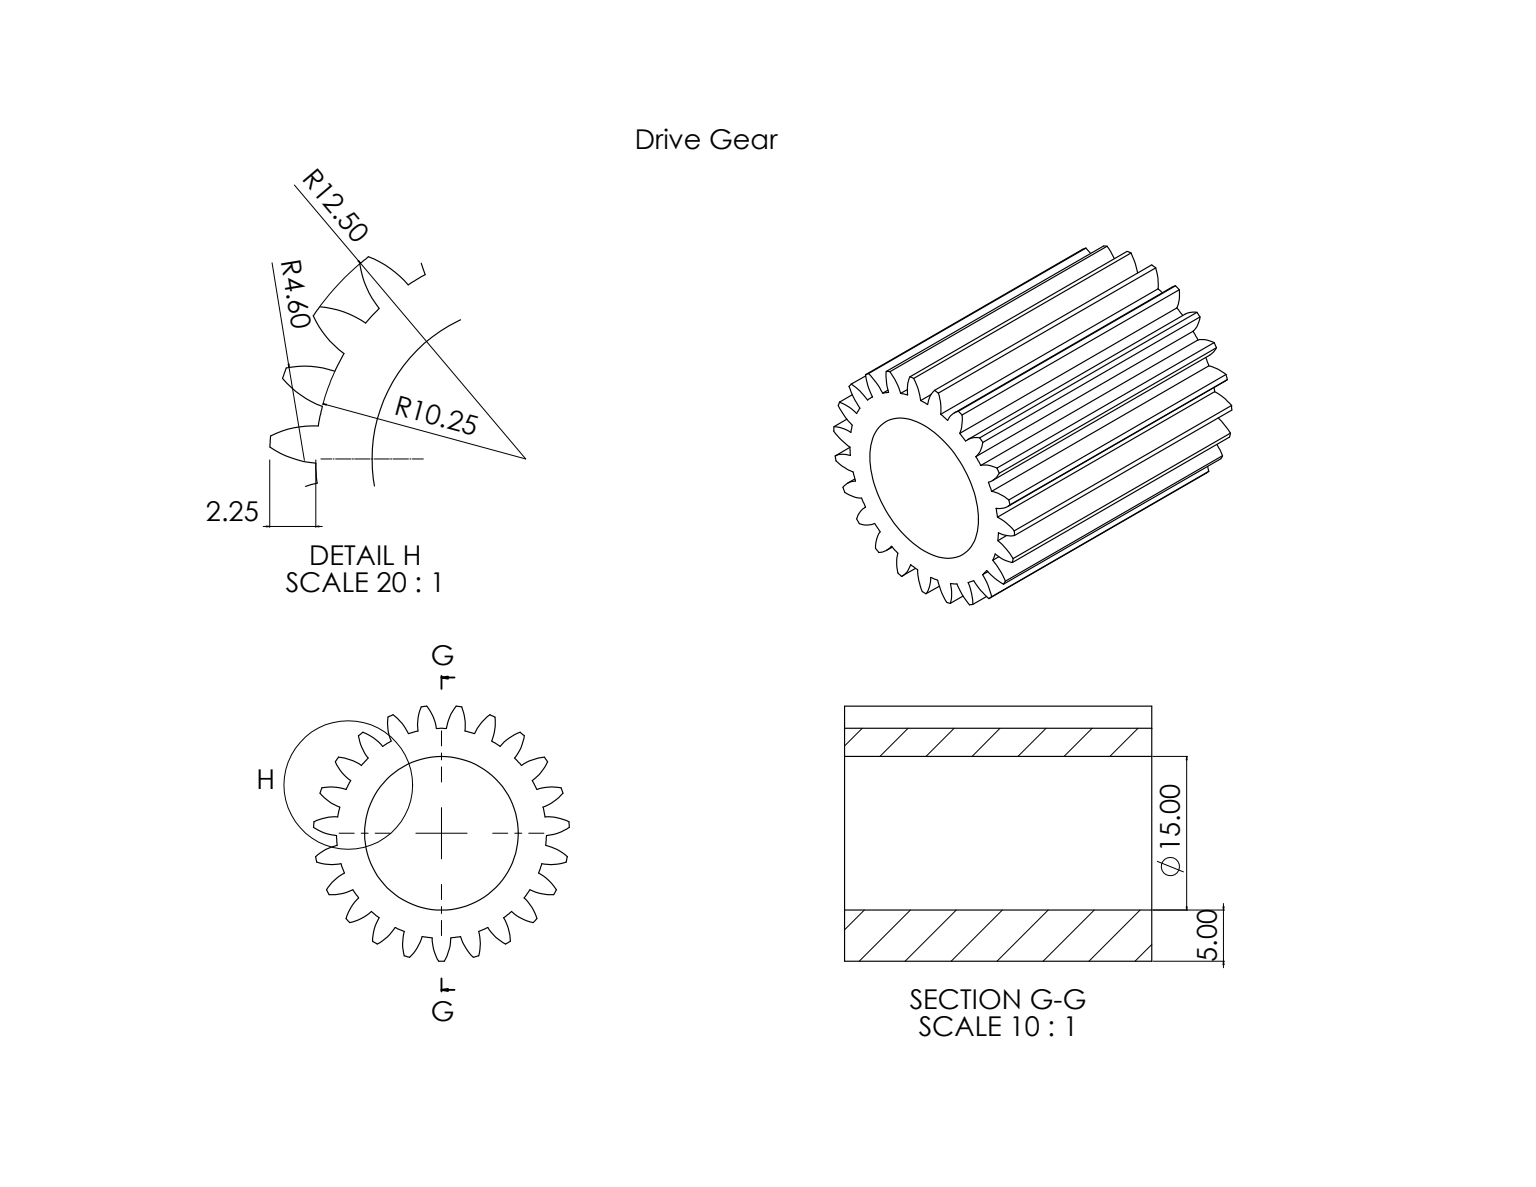
ISO-10303-21;
HEADER;
FILE_DESCRIPTION (('STEP AP214'),
    '1' );
FILE_NAME ('Drive Gear.step',
    '2026-10-21T18:33:49',
    ( '' ),
    ( '' ),
    'SwSTEP 2.0',
    'SolidWorks 2025',
    '' );
FILE_SCHEMA (( 'AUTOMOTIVE_DESIGN' ));
ENDSEC;

DATA;
#7=CIRCLE ( 'NONE', #9259, 4.600000000000006750 ) ;
#13=CIRCLE ( 'NONE', #606, 12.50000000000001776 ) ;
#15=ADVANCED_FACE ( 'NONE', ( #8489 ), #16983, .T. ) ;
#16=DIRECTION ( 'NONE',  ( -5.204170427930409450E-16, 0.000000000000000000, 1.000000000000000000 ) ) ;
#17=ORIENTED_EDGE ( 'NONE', *, *, #6060, .F. ) ;
#19=ADVANCED_FACE ( 'NONE', ( #15595 ), #11103, .T. ) ;
#20=ADVANCED_FACE ( 'NONE', ( #8576 ), #7163, .T. ) ;
#21=CARTESIAN_POINT ( 'NONE',  ( -67.50540723371459251, 87.07303407725210320, 15.00000000000006928 ) ) ;
#30=EDGE_LOOP ( 'NONE', ( #4057, #14157, #6420, #5551 ) ) ;
#37=EDGE_LOOP ( 'NONE', ( #6433, #6306, #4816, #14039 ) ) ;
#40=ORIENTED_EDGE ( 'NONE', *, *, #16480, .F. ) ;
#42=DIRECTION ( 'NONE',  ( -1.000000000000000000, 5.416250486023790304E-15, 1.692578276882434470E-16 ) ) ;
#50=ORIENTED_EDGE ( 'NONE', *, *, #8115, .F. ) ;
#51=AXIS2_PLACEMENT_3D ( 'NONE', #16170, #17306, #13379 ) ;
#53=ORIENTED_EDGE ( 'NONE', *, *, #16344, .F. ) ;
#56=AXIS2_PLACEMENT_3D ( 'NONE', #11345, #9554, #17037 ) ;
#58=DIRECTION ( 'NONE',  ( -1.000000000000000000, 0.000000000000000000, 1.156482317317869999E-16 ) ) ;
#61=CARTESIAN_POINT ( 'NONE',  ( -44.89980253466632831, 81.41924511788819530, 15.00000000000006928 ) ) ;
#62=DIRECTION ( 'NONE',  ( 1.000000000000000000, 0.000000000000000000, 5.077734830647299712E-16 ) ) ;
#70=VERTEX_POINT ( 'NONE', #417 ) ;
#71=CIRCLE ( 'NONE', #16786, 10.24900000000000055 ) ;
#72=VECTOR ( 'NONE', #8079, 1000.000000000000000 ) ;
#75=CARTESIAN_POINT ( 'NONE',  ( -59.35080917176598092, 94.79374675277695417, -15.00000000000001421 ) ) ;
#83=AXIS2_PLACEMENT_3D ( 'NONE', #305, #8649, #15842 ) ;
#86=CARTESIAN_POINT ( 'NONE',  ( -67.32681558843928826, 84.01587117655452630, 15.00000000000006928 ) ) ;
#92=FACE_OUTER_BOUND ( 'NONE', #4705, .T. ) ;
#97=EDGE_LOOP ( 'NONE', ( #14559, #13719, #17905, #14362 ) ) ;
#98=VECTOR ( 'NONE', #835, 1000.000000000000000 ) ;
#104=VECTOR ( 'NONE', #14107, 1000.000000000000000 ) ;
#113=VERTEX_POINT ( 'NONE', #1813 ) ;
#114=CARTESIAN_POINT ( 'NONE',  ( -57.08002265617300708, 84.22855780814606419, 15.00000000000006928 ) ) ;
#145=EDGE_LOOP ( 'NONE', ( #17261, #13971, #8851, #5219 ) ) ;
#147=DIRECTION ( 'NONE',  ( 1.156482317317869999E-16, 0.000000000000000000, 1.000000000000000000 ) ) ;
#149=ORIENTED_EDGE ( 'NONE', *, *, #11735, .T. ) ;
#150=EDGE_CURVE ( 'NONE', #4219, #3665, #3494, .T. ) ;
#154=AXIS2_PLACEMENT_3D ( 'NONE', #13342, #6302, #517 ) ;
#169=CARTESIAN_POINT ( 'NONE',  ( -59.35080917176598092, 94.79374675277695417, 15.00000000000006928 ) ) ;
#175=DIRECTION ( 'NONE',  ( 1.000000000000000000, 0.000000000000000000, 0.000000000000000000 ) ) ;
#179=DIRECTION ( 'NONE',  ( 1.000000000000000000, 0.000000000000000000, 5.551115123125780730E-16 ) ) ;
#187=DIRECTION ( 'NONE',  ( -5.204170427930409450E-16, 0.000000000000000000, 1.000000000000000000 ) ) ;
#191=DIRECTION ( 'NONE',  ( 1.156482317317869999E-16, 0.000000000000000000, 1.000000000000000000 ) ) ;
#195=CYLINDRICAL_SURFACE ( 'NONE', #16432, 4.599999999999999645 ) ;
#197=VERTEX_POINT ( 'NONE', #9569 ) ;
#200=ORIENTED_EDGE ( 'NONE', *, *, #18072, .T. ) ;
#201=DIRECTION ( 'NONE',  ( -1.000000000000000000, 2.331468351712825579E-14, 1.387778780781443703E-16 ) ) ;
#209=DIRECTION ( 'NONE',  ( 1.156482317317869999E-16, 0.000000000000000000, 1.000000000000000000 ) ) ;
#210=ORIENTED_EDGE ( 'NONE', *, *, #16102, .F. ) ;
#216=DIRECTION ( 'NONE',  ( 0.000000000000000000, 0.000000000000000000, 1.000000000000000000 ) ) ;
#220=ORIENTED_EDGE ( 'NONE', *, *, #11450, .F. ) ;
#237=CYLINDRICAL_SURFACE ( 'NONE', #286, 4.599999999999999645 ) ;
#249=CYLINDRICAL_SURFACE ( 'NONE', #1928, 10.24900000000000766 ) ;
#253=EDGE_LOOP ( 'NONE', ( #10457, #6808, #9246, #11912 ) ) ;
#256=DIRECTION ( 'NONE',  ( 0.000000000000000000, 0.000000000000000000, 1.000000000000000000 ) ) ;
#265=DIRECTION ( 'NONE',  ( 0.000000000000000000, 0.000000000000000000, 1.000000000000000000 ) ) ;
#272=CARTESIAN_POINT ( 'NONE',  ( -67.13262496892538422, 91.65790412808873100, -167.1454815528550739 ) ) ;
#274=VERTEX_POINT ( 'NONE', #11460 ) ;
#286=AXIS2_PLACEMENT_3D ( 'NONE', #17181, #15858, #14286 ) ;
#295=DIRECTION ( 'NONE',  ( 1.000000000000000000, 0.000000000000000000, 3.771137991253934490E-16 ) ) ;
#297=EDGE_CURVE ( 'NONE', #9307, #9072, #17170, .T. ) ;
#304=VECTOR ( 'NONE', #7741, 1000.000000000000000 ) ;
#305=CARTESIAN_POINT ( 'NONE',  ( -56.26901274438541378, 73.45256821284058901, -15.00000000000001421 ) ) ;
#309=EDGE_CURVE ( 'NONE', #9564, #16752, #11785, .T. ) ;
#311=EDGE_CURVE ( 'NONE', #17138, #8972, #12775, .T. ) ;
#319=FACE_BOUND ( 'NONE', #1203, .T. ) ;
#321=EDGE_LOOP ( 'NONE', ( #11496, #14503 ) ) ;
#328=CYLINDRICAL_SURFACE ( 'NONE', #16782, 4.599999999999999645 ) ;
#329=DIRECTION ( 'NONE',  ( 1.156482317317869999E-16, 0.000000000000000000, 1.000000000000000000 ) ) ;
#332=AXIS2_PLACEMENT_3D ( 'NONE', #14799, #4971, #14887 ) ;
#340=ADVANCED_FACE ( 'NONE', ( #13312 ), #13217, .T. ) ;
#348=CARTESIAN_POINT ( 'NONE',  ( -65.94558993203320085, 89.37090336996871542, -167.1454815528550739 ) ) ;
#351=ORIENTED_EDGE ( 'NONE', *, *, #16581, .T. ) ;
#352=DIRECTION ( 'NONE',  ( 1.000000000000000000, 0.000000000000000000, 0.000000000000000000 ) ) ;
#353=AXIS2_PLACEMENT_3D ( 'NONE', #9432, #13643, #6427 ) ;
#362=EDGE_CURVE ( 'NONE', #16861, #16195, #8816, .T. ) ;
#363=LINE ( 'NONE', #13186, #2716 ) ;
#369=ORIENTED_EDGE ( 'NONE', *, *, #4474, .F. ) ;
#370=ORIENTED_EDGE ( 'NONE', *, *, #2385, .F. ) ;
#402=AXIS2_PLACEMENT_3D ( 'NONE', #10590, #6260, #12088 ) ;
#415=VERTEX_POINT ( 'NONE', #17506 ) ;
#417=CARTESIAN_POINT ( 'NONE',  ( -50.35400969968294049, 73.69239390902568232, 15.00000000000006928 ) ) ;
#428=CARTESIAN_POINT ( 'NONE',  ( -57.08002265617300708, 84.22855780814606419, -167.1454815528550739 ) ) ;
#431=CARTESIAN_POINT ( 'NONE',  ( -67.77554565888843285, 85.77305660501664875, 15.00000000000006928 ) ) ;
#434=CIRCLE ( 'NONE', #4026, 12.50000000000001066 ) ;
#435=ORIENTED_EDGE ( 'NONE', *, *, #15098, .T. ) ;
#436=VECTOR ( 'NONE', #9546, 1000.000000000000000 ) ;
#439=CARTESIAN_POINT ( 'NONE',  ( -63.80603561266293156, 73.69239390902558284, -167.1454815528550739 ) ) ;
#440=EDGE_CURVE ( 'NONE', #16158, #9400, #4619, .T. ) ;
#445=DIRECTION ( 'NONE',  ( 0.000000000000000000, 0.000000000000000000, 1.000000000000000000 ) ) ;
#447=CIRCLE ( 'NONE', #16265, 4.599999999999999645 ) ;
#458=ORIENTED_EDGE ( 'NONE', *, *, #15095, .T. ) ;
#465=AXIS2_PLACEMENT_3D ( 'NONE', #15310, #8209, #13925 ) ;
#466=EDGE_CURVE ( 'NONE', #2633, #113, #1358, .T. ) ;
#469=EDGE_CURVE ( 'NONE', #3406, #8935, #14485, .T. ) ;
#472=DIRECTION ( 'NONE',  ( 1.000000000000000000, 0.000000000000000000, 0.000000000000000000 ) ) ;
#475=DIRECTION ( 'NONE',  ( 1.156482317317869999E-16, 0.000000000000000000, 1.000000000000000000 ) ) ;
#477=ORIENTED_EDGE ( 'NONE', *, *, #4383, .F. ) ;
#489=EDGE_CURVE ( 'NONE', #6937, #4200, #6985, .T. ) ;
#493=ORIENTED_EDGE ( 'NONE', *, *, #10731, .F. ) ;
#498=CARTESIAN_POINT ( 'NONE',  ( -57.08002265617300708, 84.22855780814606419, -15.00000000000001421 ) ) ;
#502=FACE_OUTER_BOUND ( 'NONE', #5462, .T. ) ;
#511=ORIENTED_EDGE ( 'NONE', *, *, #14433, .F. ) ;
#514=CARTESIAN_POINT ( 'NONE',  ( -57.08002265617300708, 84.22855780814606419, 15.00000000000006928 ) ) ;
#517=DIRECTION ( 'NONE',  ( -1.000000000000000000, -3.016910393003147592E-15, 0.000000000000000000 ) ) ;
#518=DIRECTION ( 'NONE',  ( 1.000000000000000000, 0.000000000000000000, 0.000000000000000000 ) ) ;
#519=ORIENTED_EDGE ( 'NONE', *, *, #11473, .F. ) ;
#522=DIRECTION ( 'NONE',  ( 0.000000000000000000, 0.000000000000000000, 1.000000000000000000 ) ) ;
#526=DIRECTION ( 'NONE',  ( 0.000000000000000000, 0.000000000000000000, 1.000000000000000000 ) ) ;
#528=EDGE_LOOP ( 'NONE', ( #8354, #7996, #14007, #17143 ) ) ;
#538=VERTEX_POINT ( 'NONE', #3755 ) ;
#539=EDGE_CURVE ( 'NONE', #1636, #14316, #3687, .T. ) ;
#544=AXIS2_PLACEMENT_3D ( 'NONE', #10480, #10583, #14958 ) ;
#548=EDGE_CURVE ( 'NONE', #15230, #8556, #6062, .T. ) ;
#563=DIRECTION ( 'NONE',  ( 0.000000000000000000, 0.000000000000000000, 1.000000000000000000 ) ) ;
#566=ADVANCED_FACE ( 'NONE', ( #8045 ), #954, .T. ) ;
#567=DIRECTION ( 'NONE',  ( 1.000000000000000000, 0.000000000000000000, 5.077734830647299712E-16 ) ) ;
#571=DIRECTION ( 'NONE',  ( 1.000000000000000000, 0.000000000000000000, 0.000000000000000000 ) ) ;
#572=DIRECTION ( 'NONE',  ( -5.204170427930409450E-16, 0.000000000000000000, 1.000000000000000000 ) ) ;
#575=VECTOR ( 'NONE', #9890, 1000.000000000000000 ) ;
#577=EDGE_CURVE ( 'NONE', #10391, #5674, #7997, .T. ) ;
#578=ORIENTED_EDGE ( 'NONE', *, *, #6429, .T. ) ;
#579=CARTESIAN_POINT ( 'NONE',  ( -69.52933024547458274, 85.35316464920589397, -15.00000000000001421 ) ) ;
#580=FACE_OUTER_BOUND ( 'NONE', #1981, .T. ) ;
#583=VERTEX_POINT ( 'NONE', #16183 ) ;
#601=DIRECTION ( 'NONE',  ( 1.156482317317869999E-16, 0.000000000000000000, 1.000000000000000000 ) ) ;
#605=ORIENTED_EDGE ( 'NONE', *, *, #15039, .T. ) ;
#606=AXIS2_PLACEMENT_3D ( 'NONE', #17023, #8618, #18357 ) ;
#616=VERTEX_POINT ( 'NONE', #17966 ) ;
#624=CARTESIAN_POINT ( 'NONE',  ( -66.02736529514692165, 75.49957964911740760, -167.1454815528550739 ) ) ;
#626=VERTEX_POINT ( 'NONE', #9934 ) ;
#630=DIRECTION ( 'NONE',  ( 0.000000000000000000, 0.000000000000000000, 1.000000000000000000 ) ) ;
#635=VECTOR ( 'NONE', #5666, 1000.000000000000000 ) ;
#643=ORIENTED_EDGE ( 'NONE', *, *, #17487, .T. ) ;
#644=AXIS2_PLACEMENT_3D ( 'NONE', #13035, #12849, #9845 ) ;
#648=DIRECTION ( 'NONE',  ( -5.204170427930409450E-16, 0.000000000000000000, 1.000000000000000000 ) ) ;
#654=ORIENTED_EDGE ( 'NONE', *, *, #15337, .F. ) ;
#659=AXIS2_PLACEMENT_3D ( 'NONE', #1736, #329, #11753 ) ;
#666=AXIS2_PLACEMENT_3D ( 'NONE', #5456, #2751, #8462 ) ;
#667=CARTESIAN_POINT ( 'NONE',  ( -66.96222586426215173, 88.60139997190893268, -15.00000000000001421 ) ) ;
#669=CARTESIAN_POINT ( 'NONE',  ( -67.26033723204500347, 83.04399200740374454, -167.1454815528550739 ) ) ;
#673=CIRCLE ( 'NONE', #13222, 4.599999999999992539 ) ;
#683=ORIENTED_EDGE ( 'NONE', *, *, #10429, .F. ) ;
#692=VECTOR ( 'NONE', #1319, 1000.000000000000000 ) ;
#703=VERTEX_POINT ( 'NONE', #18363 ) ;
#708=CIRCLE ( 'NONE', #7867, 10.24899999999999345 ) ;
#710=DIRECTION ( 'NONE',  ( -1.000000000000000000, 0.000000000000000000, 1.692578276882434470E-16 ) ) ;
#717=EDGE_CURVE ( 'NONE', #13256, #9250, #2635, .T. ) ;
#719=AXIS2_PLACEMENT_3D ( 'NONE', #3606, #2301, #18126 ) ;
#728=CYLINDRICAL_SURFACE ( 'NONE', #10885, 4.600000000000006750 ) ;
#753=CYLINDRICAL_SURFACE ( 'NONE', #2101, 10.24900000000000055 ) ;
#766=CIRCLE ( 'NONE', #8554, 4.599999999999992539 ) ;
#768=VERTEX_POINT ( 'NONE', #8808 ) ;
#774=CARTESIAN_POINT ( 'NONE',  ( -69.56651066787533466, 84.80960611389535586, -15.00000000000001421 ) ) ;
#781=ORIENTED_EDGE ( 'NONE', *, *, #10127, .F. ) ;
#782=CARTESIAN_POINT ( 'NONE',  ( -48.13268001719898592, 75.49957964911752129, -15.00000000000001421 ) ) ;
#785=ORIENTED_EDGE ( 'NONE', *, *, #3442, .T. ) ;
#805=EDGE_LOOP ( 'NONE', ( #18504, #2083, #17066, #16197 ) ) ;
#809=EDGE_CURVE ( 'NONE', #10849, #8377, #8807, .T. ) ;
#812=( NAMED_UNIT ( * ) SI_UNIT ( $, .STERADIAN. ) SOLID_ANGLE_UNIT ( ) );
#813=LINE ( 'NONE', #6502, #11347 ) ;
#815=EDGE_CURVE ( 'NONE', #6999, #415, #2223, .T. ) ;
#821=LINE ( 'NONE', #15125, #1960 ) ;
#828=EDGE_CURVE ( 'NONE', #10611, #5567, #16268, .T. ) ;
#832=CARTESIAN_POINT ( 'NONE',  ( -63.25151023250651150, 93.09943318379590949, -15.00000000000001421 ) ) ;
#834=CARTESIAN_POINT ( 'NONE',  ( -44.63071506687145984, 85.35316464920607871, 15.00000000000009592 ) ) ;
#835=DIRECTION ( 'NONE',  ( 0.000000000000000000, 0.000000000000000000, 1.000000000000000000 ) ) ;
#840=DIRECTION ( 'NONE',  ( 0.000000000000000000, 0.000000000000000000, 1.000000000000000000 ) ) ;
#841=AXIS2_PLACEMENT_3D ( 'NONE', #6547, #3474, #17867 ) ;
#845=VERTEX_POINT ( 'NONE', #8981 ) ;
#848=VERTEX_POINT ( 'NONE', #11435 ) ;
#849=AXIS2_PLACEMENT_3D ( 'NONE', #13326, #7699, #1906 ) ;
#855=DIRECTION ( 'NONE',  ( 1.000000000000000000, 0.000000000000000000, 5.551115123125786646E-16 ) ) ;
#859=CARTESIAN_POINT ( 'NONE',  ( -50.78804881079258848, 75.44273092821050852, 15.00000000000006928 ) ) ;
#860=DIRECTION ( 'NONE',  ( 0.000000000000000000, 0.000000000000000000, 1.000000000000000000 ) ) ;
#879=DIRECTION ( 'NONE',  ( -1.000000000000000000, 0.000000000000000000, 0.000000000000000000 ) ) ;
#920=ORIENTED_EDGE ( 'NONE', *, *, #3325, .F. ) ;
#925=CARTESIAN_POINT ( 'NONE',  ( -57.08002265617300708, 84.22855780814606419, -167.1454815528550739 ) ) ;
#928=LINE ( 'NONE', #6630, #98 ) ;
#937=DIRECTION ( 'NONE',  ( -1.000000000000000000, 1.760281407957729384E-14, 1.692578276882432005E-16 ) ) ;
#944=AXIS2_PLACEMENT_3D ( 'NONE', #10386, #13473, #15913 ) ;
#947=ORIENTED_EDGE ( 'NONE', *, *, #13616, .T. ) ;
#952=EDGE_CURVE ( 'NONE', #12358, #17935, #14770, .T. ) ;
#954=CYLINDRICAL_SURFACE ( 'NONE', #402, 12.49999999999999112 ) ;
#955=CARTESIAN_POINT ( 'NONE',  ( -57.08002265617300708, 84.22855780814606419, -15.00000000000001421 ) ) ;
#958=CIRCLE ( 'NONE', #8121, 4.599999999999992539 ) ;
#959=CARTESIAN_POINT ( 'NONE',  ( -46.95762973216378811, 85.83453492254348305, -167.1454815528550739 ) ) ;
#962=CARTESIAN_POINT ( 'NONE',  ( -57.89103256796045116, 73.45256821284057480, -15.00000000000001421 ) ) ;
#967=AXIS2_PLACEMENT_3D ( 'NONE', #11022, #11220, #4101 ) ;
#968=AXIS2_PLACEMENT_3D ( 'NONE', #2909, #3074, #1413 ) ;
#972=EDGE_CURVE ( 'NONE', #13894, #9284, #1056, .T. ) ;
#973=ORIENTED_EDGE ( 'NONE', *, *, #8614, .T. ) ;
#974=AXIS2_PLACEMENT_3D ( 'NONE', #4166, #8475, #15486 ) ;
#979=DIRECTION ( 'NONE',  ( 1.000000000000000000, 0.000000000000000000, 0.000000000000000000 ) ) ;
#985=CARTESIAN_POINT ( 'NONE',  ( -53.84898691462515785, 93.95493478196527803, -167.1454815528550739 ) ) ;
#989=EDGE_CURVE ( 'NONE', #1289, #768, #13897, .T. ) ;
#999=CARTESIAN_POINT ( 'NONE',  ( -54.95363092160842911, 73.63336328296981037, -15.00000000000001421 ) ) ;
#1000=VERTEX_POINT ( 'NONE', #5126 ) ;
#1002=AXIS2_PLACEMENT_3D ( 'NONE', #14462, #1461, #10148 ) ;
#1014=AXIS2_PLACEMENT_3D ( 'NONE', #667, #4964, #5050 ) ;
#1024=VERTEX_POINT ( 'NONE', #834 ) ;
#1025=EDGE_CURVE ( 'NONE', #16752, #1935, #2548, .T. ) ;
#1035=CIRCLE ( 'NONE', #6718, 10.24900000000000055 ) ;
#1042=EDGE_CURVE ( 'NONE', #9640, #3596, #2530, .T. ) ;
#1045=VERTEX_POINT ( 'NONE', #13291 ) ;
#1051=AXIS2_PLACEMENT_3D ( 'NONE', #2696, #6904, #5499 ) ;
#1056=CIRCLE ( 'NONE', #11519, 10.24900000000000055 ) ;
#1060=CARTESIAN_POINT ( 'NONE',  ( -57.08002265617300708, 84.22855780814606419, -15.00000000000001421 ) ) ;
#1073=AXIS2_PLACEMENT_3D ( 'NONE', #12166, #16356, #2049 ) ;
#1085=DIRECTION ( 'NONE',  ( -1.000000000000000000, 6.033820786006277040E-15, 0.000000000000000000 ) ) ;
#1100=ORIENTED_EDGE ( 'NONE', *, *, #2868, .T. ) ;
#1102=DIRECTION ( 'NONE',  ( 1.000000000000000000, 0.000000000000000000, 5.077734830647306615E-16 ) ) ;
#1109=ORIENTED_EDGE ( 'NONE', *, *, #1727, .T. ) ;
#1117=FACE_OUTER_BOUND ( 'NONE', #1125, .T. ) ;
#1118=CARTESIAN_POINT ( 'NONE',  ( -57.08002265617300708, 84.22855780814606419, -15.00000000000001421 ) ) ;
#1120=ORIENTED_EDGE ( 'NONE', *, *, #8674, .T. ) ;
#1125=EDGE_LOOP ( 'NONE', ( #16868, #13231, #10617, #17298 ) ) ;
#1130=ADVANCED_FACE ( 'NONE', ( #18043 ), #13938, .T. ) ;
#1131=DIRECTION ( 'NONE',  ( 1.156482317317869999E-16, 0.000000000000000000, 1.000000000000000000 ) ) ;
#1139=ORIENTED_EDGE ( 'NONE', *, *, #4989, .F. ) ;
#1147=ORIENTED_EDGE ( 'NONE', *, *, #13705, .T. ) ;
#1148=EDGE_CURVE ( 'NONE', #15468, #8935, #14128, .T. ) ;
#1149=DIRECTION ( 'NONE',  ( -1.000000000000000000, 0.000000000000000000, 0.000000000000000000 ) ) ;
#1152=ORIENTED_EDGE ( 'NONE', *, *, #311, .T. ) ;
#1164=AXIS2_PLACEMENT_3D ( 'NONE', #3751, #12553, #6745 ) ;
#1171=LINE ( 'NONE', #5559, #1945 ) ;
#1184=CARTESIAN_POINT ( 'NONE',  ( -48.98198201484814263, 93.75072866207695199, -167.1454815528550739 ) ) ;
#1185=ORIENTED_EDGE ( 'NONE', *, *, #12268, .T. ) ;
#1187=VERTEX_POINT ( 'NONE', #17461 ) ;
#1192=CARTESIAN_POINT ( 'NONE',  ( -53.44817431141344599, 74.64462966772957486, -167.1454815528550739 ) ) ;
#1198=VECTOR ( 'NONE', #8394, 1000.000000000000000 ) ;
#1199=DIRECTION ( 'NONE',  ( 1.000000000000000000, 0.000000000000000000, 0.000000000000000000 ) ) ;
#1203=EDGE_LOOP ( 'NONE', ( #7524, #14271 ) ) ;
#1206=DIRECTION ( 'NONE',  ( -1.000000000000000000, 0.000000000000000000, 0.000000000000000000 ) ) ;
#1209=VECTOR ( 'NONE', #18271, 1000.000000000000000 ) ;
#1220=DIRECTION ( 'NONE',  ( 0.000000000000000000, 0.000000000000000000, 1.000000000000000000 ) ) ;
#1229=DIRECTION ( 'NONE',  ( 1.156482317317869999E-16, 0.000000000000000000, 1.000000000000000000 ) ) ;
#1231=VERTEX_POINT ( 'NONE', #8604 ) ;
#1234=ORIENTED_EDGE ( 'NONE', *, *, #5956, .F. ) ;
#1235=UNCERTAINTY_MEASURE_WITH_UNIT (LENGTH_MEASURE( 1.000000000000000082E-05 ), #17113, 'distance_accuracy_value', 'NONE');
#1236=CIRCLE ( 'NONE', #7215, 10.24900000000000055 ) ;
#1249=ADVANCED_FACE ( 'NONE', ( #3068 ), #14305, .T. ) ;
#1254=ORIENTED_EDGE ( 'NONE', *, *, #4048, .T. ) ;
#1256=ADVANCED_FACE ( 'NONE', ( #15793 ), #17278, .T. ) ;
#1262=AXIS2_PLACEMENT_3D ( 'NONE', #1972, #10573, #13375 ) ;
#1265=ORIENTED_EDGE ( 'NONE', *, *, #2637, .F. ) ;
#1274=ORIENTED_EDGE ( 'NONE', *, *, #4335, .T. ) ;
#1280=AXIS2_PLACEMENT_3D ( 'NONE', #10908, #15287, #15186 ) ;
#1282=ORIENTED_EDGE ( 'NONE', *, *, #15902, .F. ) ;
#1283=ADVANCED_FACE ( 'NONE', ( #14742 ), #14917, .T. ) ;
#1289=VERTEX_POINT ( 'NONE', #7923 ) ;
#1290=EDGE_CURVE ( 'NONE', #415, #13190, #3329, .T. ) ;
#1291=CARTESIAN_POINT ( 'NONE',  ( -69.26024277767963611, 81.41924511788803898, -15.00000000000001243 ) ) ;
#1294=DIRECTION ( 'NONE',  ( -5.204170427930409450E-16, 0.000000000000000000, 1.000000000000000000 ) ) ;
#1298=VECTOR ( 'NONE', #12416, 1000.000000000000000 ) ;
#1299=AXIS2_PLACEMENT_3D ( 'NONE', #11088, #17069, #11190 ) ;
#1301=DIRECTION ( 'NONE',  ( -5.204170427930409450E-16, 0.000000000000000000, 1.000000000000000000 ) ) ;
#1304=ADVANCED_FACE ( 'NONE', ( #2020 ), #13538, .T. ) ;
#1308=AXIS2_PLACEMENT_3D ( 'NONE', #1669, #8784, #9145 ) ;
#1311=ORIENTED_EDGE ( 'NONE', *, *, #8334, .F. ) ;
#1319=DIRECTION ( 'NONE',  ( 0.000000000000000000, 0.000000000000000000, 1.000000000000000000 ) ) ;
#1320=CARTESIAN_POINT ( 'NONE',  ( -53.97067643794850511, 72.12145385653101926, -15.00000000000001421 ) ) ;
#1338=AXIS2_PLACEMENT_3D ( 'NONE', #3757, #8048, #13769 ) ;
#1343=LINE ( 'NONE', #5627, #9553 ) ;
#1349=LINE ( 'NONE', #7056, #7856 ) ;
#1353=VECTOR ( 'NONE', #15756, 1000.000000000000000 ) ;
#1358=CIRCLE ( 'NONE', #13587, 4.599999999999999645 ) ;
#1374=ORIENTED_EDGE ( 'NONE', *, *, #1830, .T. ) ;
#1375=ADVANCED_FACE ( 'NONE', ( #13438 ), #10361, .T. ) ;
#1381=EDGE_CURVE ( 'NONE', #14903, #12673, #14655, .T. ) ;
#1386=CARTESIAN_POINT ( 'NONE',  ( -55.20348911625212907, 74.15281352429526862, 15.00000000000006928 ) ) ;
#1394=ADVANCED_FACE ( 'NONE', ( #16930 ), #4117, .T. ) ;
#1399=VERTEX_POINT ( 'NONE', #10846 ) ;
#1400=ORIENTED_EDGE ( 'NONE', *, *, #17950, .F. ) ;
#1403=CYLINDRICAL_SURFACE ( 'NONE', #8481, 4.600000000000006750 ) ;
#1413=DIRECTION ( 'NONE',  ( 1.000000000000000000, 0.000000000000000000, 0.000000000000000000 ) ) ;
#1414=ORIENTED_EDGE ( 'NONE', *, *, #17886, .T. ) ;
#1416=LINE ( 'NONE', #18355, #18244 ) ;
#1417=EDGE_LOOP ( 'NONE', ( #13121, #10077, #10249, #16577 ) ) ;
#1419=CARTESIAN_POINT ( 'NONE',  ( -57.08002265617300708, 84.22855780814606419, 15.00000000000006928 ) ) ;
#1421=ORIENTED_EDGE ( 'NONE', *, *, #16791, .T. ) ;
#1424=DIRECTION ( 'NONE',  ( -1.000000000000000000, 2.442490654175343758E-14, 1.387778780781445182E-16 ) ) ;
#1437=ADVANCED_FACE ( 'NONE', ( #8030 ), #15235, .T. ) ;
#1439=CARTESIAN_POINT ( 'NONE',  ( -60.76828531927866095, 74.07097899412299569, -15.00000000000001421 ) ) ;
#1448=AXIS2_PLACEMENT_3D ( 'NONE', #16760, #3769, #10887 ) ;
#1450=CARTESIAN_POINT ( 'NONE',  ( -57.08002265617300708, 84.22855780814606419, -167.1454815528550739 ) ) ;
#1451=DIRECTION ( 'NONE',  ( 0.000000000000000000, 0.000000000000000000, 1.000000000000000000 ) ) ;
#1461=DIRECTION ( 'NONE',  ( 0.000000000000000000, 0.000000000000000000, 1.000000000000000000 ) ) ;
#1472=ORIENTED_EDGE ( 'NONE', *, *, #9755, .T. ) ;
#1473=DIRECTION ( 'NONE',  ( -5.204170427930409450E-16, 0.000000000000000000, 1.000000000000000000 ) ) ;
#1476=CARTESIAN_POINT ( 'NONE',  ( -52.17393402261416213, 74.59995546124159205, -167.1454815528550739 ) ) ;
#1481=DIRECTION ( 'NONE',  ( 1.156482317317869999E-16, 0.000000000000000000, 1.000000000000000000 ) ) ;
#1488=ORIENTED_EDGE ( 'NONE', *, *, #12791, .T. ) ;
#1496=AXIS2_PLACEMENT_3D ( 'NONE', #8750, #14455, #1638 ) ;
#1497=EDGE_CURVE ( 'NONE', #2307, #10454, #14495, .T. ) ;
#1498=ORIENTED_EDGE ( 'NONE', *, *, #17806, .T. ) ;
#1505=ADVANCED_FACE ( 'NONE', ( #3073 ), #5603, .T. ) ;
#1513=CYLINDRICAL_SURFACE ( 'NONE', #8051, 4.599999999999992539 ) ;
#1517=ORIENTED_EDGE ( 'NONE', *, *, #12616, .T. ) ;
#1523=AXIS2_PLACEMENT_3D ( 'NONE', #13994, #2279, #16596 ) ;
#1524=DIRECTION ( 'NONE',  ( 0.000000000000000000, 0.000000000000000000, 1.000000000000000000 ) ) ;
#1525=EDGE_CURVE ( 'NONE', #10995, #13256, #5846, .T. ) ;
#1529=CIRCLE ( 'NONE', #11967, 4.599999999999999645 ) ;
#1532=DIRECTION ( 'NONE',  ( -5.204170427930409450E-16, 0.000000000000000000, 1.000000000000000000 ) ) ;
#1539=CYLINDRICAL_SURFACE ( 'NONE', #2742, 12.50000000000001776 ) ;
#1542=ORIENTED_EDGE ( 'NONE', *, *, #14644, .T. ) ;
#1548=AXIS2_PLACEMENT_3D ( 'NONE', #12923, #5789, #3250 ) ;
#1560=DIRECTION ( 'NONE',  ( 0.000000000000000000, 0.000000000000000000, 1.000000000000000000 ) ) ;
#1562=VERTEX_POINT ( 'NONE', #11595 ) ;
#1563=EDGE_CURVE ( 'NONE', #11670, #2929, #1579, .T. ) ;
#1579=LINE ( 'NONE', #5875, #12744 ) ;
#1586=ORIENTED_EDGE ( 'NONE', *, *, #10900, .F. ) ;
#1590=AXIS2_PLACEMENT_3D ( 'NONE', #6597, #3600, #13810 ) ;
#1592=ORIENTED_EDGE ( 'NONE', *, *, #362, .T. ) ;
#1598=DIRECTION ( 'NONE',  ( -5.204170427930409450E-16, 0.000000000000000000, 1.000000000000000000 ) ) ;
#1600=CARTESIAN_POINT ( 'NONE',  ( -67.44681693414594292, 91.21279551874751235, -167.1454815528550739 ) ) ;
#1601=EDGE_CURVE ( 'NONE', #12783, #14981, #4357, .T. ) ;
#1604=AXIS2_PLACEMENT_3D ( 'NONE', #7164, #17432, #58 ) ;
#1607=CARTESIAN_POINT ( 'NONE',  ( -55.10846673861666289, 96.57209730311868157, -15.00000000000001421 ) ) ;
#1610=LINE ( 'NONE', #10211, #4762 ) ;
#1612=EDGE_CURVE ( 'NONE', #1562, #14366, #7338, .T. ) ;
#1623=CARTESIAN_POINT ( 'NONE',  ( -57.08002265617300708, 84.22855780814606419, -167.1454815528550739 ) ) ;
#1636=VERTEX_POINT ( 'NONE', #10725 ) ;
#1638=DIRECTION ( 'NONE',  ( 1.000000000000000000, 0.000000000000000000, 0.000000000000000000 ) ) ;
#1643=ORIENTED_EDGE ( 'NONE', *, *, #15148, .T. ) ;
#1656=VERTEX_POINT ( 'NONE', #12146 ) ;
#1659=CARTESIAN_POINT ( 'NONE',  ( -57.08002265617300708, 84.22855780814606419, -167.1454815528550739 ) ) ;
#1667=AXIS2_PLACEMENT_3D ( 'NONE', #16475, #7969, #17976 ) ;
#1669=CARTESIAN_POINT ( 'NONE',  ( -60.62932119839002354, 94.43552448259767118, -15.00000000000001421 ) ) ;
#1679=ORIENTED_EDGE ( 'NONE', *, *, #6527, .F. ) ;
#1695=CARTESIAN_POINT ( 'NONE',  ( -66.39923980726636898, 75.89776002577445979, -15.00000000000001421 ) ) ;
#1698=CARTESIAN_POINT ( 'NONE',  ( -56.16856596726385220, 74.02016676429185793, -167.1454815528550739 ) ) ;
#1701=ORIENTED_EDGE ( 'NONE', *, *, #11701, .F. ) ;
#1720=EDGE_CURVE ( 'NONE', #10424, #16418, #14506, .T. ) ;
#1725=ADVANCED_FACE ( 'NONE', ( #15419 ), #15211, .T. ) ;
#1726=EDGE_LOOP ( 'NONE', ( #5270, #13430, #4448, #13516 ) ) ;
#1727=EDGE_CURVE ( 'NONE', #5292, #11248, #17479, .T. ) ;
#1728=ADVANCED_FACE ( 'NONE', ( #7932 ), #14014, .T. ) ;
#1736=CARTESIAN_POINT ( 'NONE',  ( -57.08002265617300708, 84.22855780814606419, -15.00000000000001421 ) ) ;
#1739=CIRCLE ( 'NONE', #11889, 4.599999999999992539 ) ;
#1754=CARTESIAN_POINT ( 'NONE',  ( -59.37303238940180705, 94.21775734381046163, -167.1454815528550739 ) ) ;
#1766=AXIS2_PLACEMENT_3D ( 'NONE', #11702, #7394, #17033 ) ;
#1767=ORIENTED_EDGE ( 'NONE', *, *, #6616, .T. ) ;
#1768=ORIENTED_EDGE ( 'NONE', *, *, #6527, .T. ) ;
#1770=CARTESIAN_POINT ( 'NONE',  ( -57.08002265617300708, 84.22855780814606419, -15.00000000000001421 ) ) ;
#1786=ORIENTED_EDGE ( 'NONE', *, *, #13989, .T. ) ;
#1794=ORIENTED_EDGE ( 'NONE', *, *, #6396, .T. ) ;
#1795=EDGE_LOOP ( 'NONE', ( #10974, #9798, #1882, #12578 ) ) ;
#1799=CIRCLE ( 'NONE', #2107, 10.24900000000001477 ) ;
#1808=ORIENTED_EDGE ( 'NONE', *, *, #989, .T. ) ;
#1813=CARTESIAN_POINT ( 'NONE',  ( -63.80603561266293156, 73.69239390902558284, 15.00000000000006928 ) ) ;
#1819=FACE_OUTER_BOUND ( 'NONE', #3573, .T. ) ;
#1820=EDGE_CURVE ( 'NONE', #11538, #12358, #18096, .T. ) ;
#1825=CARTESIAN_POINT ( 'NONE',  ( -57.08002265617300708, 84.22855780814606419, -15.00000000000001421 ) ) ;
#1826=CYLINDRICAL_SURFACE ( 'NONE', #4828, 12.49999999999999112 ) ;
#1830=EDGE_CURVE ( 'NONE', #16012, #583, #766, .T. ) ;
#1831=EDGE_CURVE ( 'NONE', #2137, #11848, #17201, .T. ) ;
#1832=DIRECTION ( 'NONE',  ( 0.000000000000000000, 0.000000000000000000, 1.000000000000000000 ) ) ;
#1844=CARTESIAN_POINT ( 'NONE',  ( -69.26024277767963611, 81.41924511788803898, -167.1454815528550739 ) ) ;
#1845=DIRECTION ( 'NONE',  ( -1.000000000000000000, -3.016910393003142859E-15, 0.000000000000000000 ) ) ;
#1856=CARTESIAN_POINT ( 'NONE',  ( -46.65463807863145007, 87.07303407725225952, 15.00000000000009592 ) ) ;
#1861=CARTESIAN_POINT ( 'NONE',  ( -56.26901274438541378, 73.45256821284058901, -167.1454815528550739 ) ) ;
#1865=CIRCLE ( 'NONE', #16187, 10.24900000000000055 ) ;
#1870=LINE ( 'NONE', #7578, #15513 ) ;
#1880=CIRCLE ( 'NONE', #12348, 4.600000000000006750 ) ;
#1882=ORIENTED_EDGE ( 'NONE', *, *, #3103, .T. ) ;
#1889=AXIS2_PLACEMENT_3D ( 'NONE', #2431, #2534, #6639 ) ;
#1898=DIRECTION ( 'NONE',  ( 1.156482317317869999E-16, 0.000000000000000000, 1.000000000000000000 ) ) ;
#1903=ORIENTED_EDGE ( 'NONE', *, *, #2637, .T. ) ;
#1906=DIRECTION ( 'NONE',  ( 1.000000000000000000, 0.000000000000000000, 0.000000000000000000 ) ) ;
#1912=CARTESIAN_POINT ( 'NONE',  ( -63.91856434051376823, 76.59466308582156557, -15.00000000000001421 ) ) ;
#1913=ORIENTED_EDGE ( 'NONE', *, *, #309, .T. ) ;
#1928=AXIS2_PLACEMENT_3D ( 'NONE', #1659, #15962, #175 ) ;
#1931=VERTEX_POINT ( 'NONE', #4098 ) ;
#1933=EDGE_CURVE ( 'NONE', #9072, #9564, #8852, .T. ) ;
#1934=ORIENTED_EDGE ( 'NONE', *, *, #17501, .F. ) ;
#1935=VERTEX_POINT ( 'NONE', #7415 ) ;
#1936=LINE ( 'NONE', #2295, #12978 ) ;
#1937=DIRECTION ( 'NONE',  ( 1.000000000000000000, 0.000000000000000000, 0.000000000000000000 ) ) ;
#1945=VECTOR ( 'NONE', #18289, 1000.000000000000000 ) ;
#1946=DIRECTION ( 'NONE',  ( 1.000000000000000000, 0.000000000000000000, 5.077734830647302671E-16 ) ) ;
#1960=VECTOR ( 'NONE', #12148, 1000.000000000000000 ) ;
#1972=CARTESIAN_POINT ( 'NONE',  ( -65.50906076758114693, 77.46608744949911340, -167.1454815528550739 ) ) ;
#1980=FACE_OUTER_BOUND ( 'NONE', #6155, .T. ) ;
#1981=EDGE_LOOP ( 'NONE', ( #8847, #9057, #17581, #5148 ) ) ;
#1982=EDGE_CURVE ( 'NONE', #12444, #4498, #4897, .T. ) ;
#1985=CYLINDRICAL_SURFACE ( 'NONE', #2205, 10.24900000000000055 ) ;
#1993=ORIENTED_EDGE ( 'NONE', *, *, #3552, .F. ) ;
#1998=ORIENTED_EDGE ( 'NONE', *, *, #12791, .F. ) ;
#2005=ORIENTED_EDGE ( 'NONE', *, *, #9619, .F. ) ;
#2011=VERTEX_POINT ( 'NONE', #13402 ) ;
#2016=DIRECTION ( 'NONE',  ( 0.000000000000000000, 0.000000000000000000, 1.000000000000000000 ) ) ;
#2018=VERTEX_POINT ( 'NONE', #15078 ) ;
#2019=PRODUCT_CONTEXT ( 'NONE', #3944, 'mechanical' ) ;
#2020=FACE_OUTER_BOUND ( 'NONE', #5279, .T. ) ;
#2021=( LENGTH_UNIT ( ) NAMED_UNIT ( * ) SI_UNIT ( .MILLI., .METRE. ) );
#2038=LINE ( 'NONE', #272, #304 ) ;
#2039=ORIENTED_EDGE ( 'NONE', *, *, #17075, .T. ) ;
#2040=VERTEX_POINT ( 'NONE', #16297 ) ;
#2041=EDGE_CURVE ( 'NONE', #7016, #17935, #10603, .T. ) ;
#2046=CARTESIAN_POINT ( 'NONE',  ( -52.35105328106566702, 95.79950628479642205, -167.1454815528550739 ) ) ;
#2049=DIRECTION ( 'NONE',  ( 1.000000000000000000, 0.000000000000000000, 5.551115123125784674E-16 ) ) ;
#2050=DIRECTION ( 'NONE',  ( 0.000000000000000000, 0.000000000000000000, 1.000000000000000000 ) ) ;
#2083=ORIENTED_EDGE ( 'NONE', *, *, #3300, .T. ) ;
#2091=AXIS2_PLACEMENT_3D ( 'NONE', #15772, #2957, #12888 ) ;
#2101=AXIS2_PLACEMENT_3D ( 'NONE', #9531, #7851, #3826 ) ;
#2103=DIRECTION ( 'NONE',  ( 0.000000000000000000, 0.000000000000000000, 1.000000000000000000 ) ) ;
#2104=CARTESIAN_POINT ( 'NONE',  ( -57.08002265617300708, 84.22855780814606419, -15.00000000000001421 ) ) ;
#2105=ORIENTED_EDGE ( 'NONE', *, *, #7355, .T. ) ;
#2107=AXIS2_PLACEMENT_3D ( 'NONE', #11691, #17379, #16342 ) ;
#2112=DIRECTION ( 'NONE',  ( -1.000000000000000000, 3.114344029463675185E-14, 1.692578276882432005E-16 ) ) ;
#2114=DIRECTION ( 'NONE',  ( -5.204170427930409450E-16, 0.000000000000000000, 1.000000000000000000 ) ) ;
#2117=LINE ( 'NONE', #10720, #17712 ) ;
#2123=CARTESIAN_POINT ( 'NONE',  ( -57.08002265617300708, 84.22855780814606419, -167.1454815528550739 ) ) ;
#2126=AXIS2_PLACEMENT_3D ( 'NONE', #9968, #4514, #2862 ) ;
#2131=CARTESIAN_POINT ( 'NONE',  ( -68.30128029835485393, 78.72098330317788850, -167.1454815528550739 ) ) ;
#2135=AXIS2_PLACEMENT_3D ( 'NONE', #962, #18080, #1149 ) ;
#2137=VERTEX_POINT ( 'NONE', #10839 ) ;
#2143=DIRECTION ( 'NONE',  ( 1.000000000000000000, 0.000000000000000000, 0.000000000000000000 ) ) ;
#2147=LINE ( 'NONE', #6829, #4780 ) ;
#2170=ADVANCED_FACE ( 'NONE', ( #14852 ), #3734, .T. ) ;
#2171=DIRECTION ( 'NONE',  ( -5.204170427930409450E-16, 0.000000000000000000, 1.000000000000000000 ) ) ;
#2175=CIRCLE ( 'NONE', #10243, 12.49999999999999112 ) ;
#2178=EDGE_CURVE ( 'NONE', #15057, #6937, #11751, .T. ) ;
#2190=DIRECTION ( 'NONE',  ( 1.000000000000000000, 0.000000000000000000, 3.771137991253928573E-16 ) ) ;
#2203=ORIENTED_EDGE ( 'NONE', *, *, #8507, .T. ) ;
#2205=AXIS2_PLACEMENT_3D ( 'NONE', #13488, #9278, #571 ) ;
#2206=ORIENTED_EDGE ( 'NONE', *, *, #17842, .T. ) ;
#2218=CARTESIAN_POINT ( 'NONE',  ( -57.08002265617300708, 84.22855780814606419, -167.1454815528550739 ) ) ;
#2220=ORIENTED_EDGE ( 'NONE', *, *, #10741, .F. ) ;
#2223=CIRCLE ( 'NONE', #7309, 12.50000000000001776 ) ;
#2226=EDGE_LOOP ( 'NONE', ( #3857, #16310, #14901, #4681 ) ) ;
#2242=DIRECTION ( 'NONE',  ( 1.000000000000000000, 0.000000000000000000, 3.771137991253934490E-16 ) ) ;
#2243=FACE_OUTER_BOUND ( 'NONE', #17880, .T. ) ;
#2246=CARTESIAN_POINT ( 'NONE',  ( -49.40461175531926585, 94.09456345901895702, -167.1454815528550739 ) ) ;
#2251=( GEOMETRIC_REPRESENTATION_CONTEXT ( 3 ) GLOBAL_UNCERTAINTY_ASSIGNED_CONTEXT ( ( #1235 ) ) GLOBAL_UNIT_ASSIGNED_CONTEXT ( ( #17113, #10019, #12920 ) ) REPRESENTATION_CONTEXT ( 'NONE', 'WORKASPACE' ) );
#2255=EDGE_CURVE ( 'NONE', #13790, #1045, #16822, .T. ) ;
#2262=ORIENTED_EDGE ( 'NONE', *, *, #6058, .F. ) ;
#2266=DIRECTION ( 'NONE',  ( 1.000000000000000000, 0.000000000000000000, 3.771137991253934490E-16 ) ) ;
#2271=VERTEX_POINT ( 'NONE', #16824 ) ;
#2279=DIRECTION ( 'NONE',  ( -5.204170427930409450E-16, 0.000000000000000000, 1.000000000000000000 ) ) ;
#2282=ORIENTED_EDGE ( 'NONE', *, *, #11444, .T. ) ;
#2283=EDGE_CURVE ( 'NONE', #14959, #8437, #16516, .T. ) ;
#2288=ADVANCED_FACE ( 'NONE', ( #6816 ), #1403, .T. ) ;
#2295=CARTESIAN_POINT ( 'NONE',  ( -64.22944241949029731, 91.57211267264378307, -167.1454815528550739 ) ) ;
#2296=CARTESIAN_POINT ( 'NONE',  ( -50.99714023269321217, 75.97988867778809663, -167.1454815528550739 ) ) ;
#2301=DIRECTION ( 'NONE',  ( 0.000000000000000000, 0.000000000000000000, 1.000000000000000000 ) ) ;
#2304=DIRECTION ( 'NONE',  ( 1.000000000000000000, 0.000000000000000000, 0.000000000000000000 ) ) ;
#2305=FACE_OUTER_BOUND ( 'NONE', #253, .T. ) ;
#2307=VERTEX_POINT ( 'NONE', #18340 ) ;
#2311=EDGE_CURVE ( 'NONE', #845, #113, #18431, .T. ) ;
#2312=ORIENTED_EDGE ( 'NONE', *, *, #2311, .F. ) ;
#2318=ADVANCED_BREP_SHAPE_REPRESENTATION ( '', ( #12580, #16217 ), #9669 ) ;
#2322=DIRECTION ( 'NONE',  ( 0.000000000000000000, 0.000000000000000000, 1.000000000000000000 ) ) ;
#2327=VERTEX_POINT ( 'NONE', #16137 ) ;
#2329=CARTESIAN_POINT ( 'NONE',  ( -57.74389692835771370, 95.01461175692088545, 15.00000000000006928 ) ) ;
#2333=ORIENTED_EDGE ( 'NONE', *, *, #16248, .T. ) ;
#2341=ADVANCED_FACE ( 'NONE', ( #8957 ), #14483, .T. ) ;
#2349=ORIENTED_EDGE ( 'NONE', *, *, #2350, .T. ) ;
#2350=EDGE_CURVE ( 'NONE', #12214, #4736, #2807, .T. ) ;
#2358=CIRCLE ( 'NONE', #16701, 4.599999999999999645 ) ;
#2360=CARTESIAN_POINT ( 'NONE',  ( -57.08002265617300708, 84.22855780814606419, 15.00000000000006928 ) ) ;
#2371=CIRCLE ( 'NONE', #5052, 10.24900000000001477 ) ;
#2382=ADVANCED_FACE ( 'NONE', ( #9050 ), #7373, .T. ) ;
#2383=CARTESIAN_POINT ( 'NONE',  ( -57.08002265617300708, 84.22855780814606419, 15.00000000000006928 ) ) ;
#2385=EDGE_CURVE ( 'NONE', #11275, #197, #10171, .T. ) ;
#2387=AXIS2_PLACEMENT_3D ( 'NONE', #12250, #17944, #5129 ) ;
#2392=CARTESIAN_POINT ( 'NONE',  ( -47.02742034342072941, 91.65790412808885890, -15.00000000000001421 ) ) ;
#2395=CARTESIAN_POINT ( 'NONE',  ( -67.88623620617454435, 84.15481808402788033, -167.1454815528550739 ) ) ;
#2401=AXIS2_PLACEMENT_3D ( 'NONE', #8513, #9810, #2699 ) ;
#2409=VECTOR ( 'NONE', #3151, 1000.000000000000000 ) ;
#2411=ORIENTED_EDGE ( 'NONE', *, *, #11467, .F. ) ;
#2412=AXIS2_PLACEMENT_3D ( 'NONE', #1476, #15613, #2894 ) ;
#2417=ORIENTED_EDGE ( 'NONE', *, *, #3676, .T. ) ;
#2424=AXIS2_PLACEMENT_3D ( 'NONE', #4444, #10157, #11493 ) ;
#2431=CARTESIAN_POINT ( 'NONE',  ( -62.11705611183893438, 93.78931001713317528, -15.00000000000001421 ) ) ;
#2449=CARTESIAN_POINT ( 'NONE',  ( -49.58002265617300708, 84.22855780814606419, -15.00000000000001421 ) ) ;
#2450=VERTEX_POINT ( 'NONE', #11851 ) ;
#2452=DIRECTION ( 'NONE',  ( 0.000000000000000000, 0.000000000000000000, 1.000000000000000000 ) ) ;
#2457=CIRCLE ( 'NONE', #4829, 12.50000000000001776 ) ;
#2468=CYLINDRICAL_SURFACE ( 'NONE', #666, 12.50000000000001066 ) ;
#2475=DIRECTION ( 'NONE',  ( 0.000000000000000000, 0.000000000000000000, 1.000000000000000000 ) ) ;
#2477=LINE ( 'NONE', #8471, #11737 ) ;
#2483=AXIS2_PLACEMENT_3D ( 'NONE', #14914, #2114, #13534 ) ;
#2485=AXIS2_PLACEMENT_3D ( 'NONE', #10357, #14738, #15875 ) ;
#2486=CARTESIAN_POINT ( 'NONE',  ( -57.99147934508202695, 74.02016676429184372, -167.1454815528550739 ) ) ;
#2489=LINE ( 'NONE', #13914, #14735 ) ;
#2493=VECTOR ( 'NONE', #17943, 1000.000000000000000 ) ;
#2496=CIRCLE ( 'NONE', #16231, 10.24900000000001477 ) ;
#2511=CIRCLE ( 'NONE', #3388, 12.49999999999999112 ) ;
#2513=CIRCLE ( 'NONE', #1338, 10.24899999999999345 ) ;
#2517=ORIENTED_EDGE ( 'NONE', *, *, #5620, .T. ) ;
#2522=ORIENTED_EDGE ( 'NONE', *, *, #8591, .T. ) ;
#2523=VECTOR ( 'NONE', #12420, 1000.000000000000000 ) ;
#2530=CIRCLE ( 'NONE', #13002, 10.24899999999998812 ) ;
#2532=PRODUCT ( 'Drive Gear', 'Drive Gear', '', ( #2019 ) ) ;
#2534=DIRECTION ( 'NONE',  ( 1.156482317317869999E-16, 0.000000000000000000, 1.000000000000000000 ) ) ;
#2536=DIRECTION ( 'NONE',  ( -5.204170427930409450E-16, 0.000000000000000000, 1.000000000000000000 ) ) ;
#2548=CIRCLE ( 'NONE', #7032, 10.24899999999998812 ) ;
#2551=ADVANCED_FACE ( 'NONE', ( #15115 ), #9319, .T. ) ;
#2552=EDGE_CURVE ( 'NONE', #14168, #3406, #1936, .T. ) ;
#2557=DIRECTION ( 'NONE',  ( 1.156482317317869999E-16, 0.000000000000000000, 1.000000000000000000 ) ) ;
#2560=CIRCLE ( 'NONE', #18079, 4.600000000000020961 ) ;
#2568=ORIENTED_EDGE ( 'NONE', *, *, #1290, .T. ) ;
#2569=CARTESIAN_POINT ( 'NONE',  ( -52.55467279550843784, 75.03273214436886462, 15.00000000000006928 ) ) ;
#2583=DIRECTION ( 'NONE',  ( 0.000000000000000000, 0.000000000000000000, 1.000000000000000000 ) ) ;
#2585=ORIENTED_EDGE ( 'NONE', *, *, #17243, .T. ) ;
#2596=EDGE_LOOP ( 'NONE', ( #4401, #6883, #8878, #2682 ) ) ;
#2604=DIRECTION ( 'NONE',  ( -5.204170427930409450E-16, 0.000000000000000000, 1.000000000000000000 ) ) ;
#2616=ORIENTED_EDGE ( 'NONE', *, *, #11228, .F. ) ;
#2623=DIRECTION ( 'NONE',  ( 1.000000000000000000, 0.000000000000000000, 0.000000000000000000 ) ) ;
#2624=CARTESIAN_POINT ( 'NONE',  ( -57.08002265617300708, 84.22855780814606419, 15.00000000000006928 ) ) ;
#2629=FACE_OUTER_BOUND ( 'NONE', #18193, .T. ) ;
#2633=VERTEX_POINT ( 'NONE', #9140 ) ;
#2634=ADVANCED_FACE ( 'NONE', ( #14828 ), #13432, .T. ) ;
#2635=LINE ( 'NONE', #3841, #436 ) ;
#2637=EDGE_CURVE ( 'NONE', #3659, #616, #2496, .T. ) ;
#2641=CARTESIAN_POINT ( 'NONE',  ( -50.81952187608693805, 73.40930968350535579, -167.1454815528550739 ) ) ;
#2646=DIRECTION ( 'NONE',  ( -1.000000000000000000, -1.218656359355351063E-14, 1.692578276882432005E-16 ) ) ;
#2650=EDGE_CURVE ( 'NONE', #3838, #3665, #16533, .T. ) ;
#2652=EDGE_CURVE ( 'NONE', #2688, #14160, #2489, .T. ) ;
#2655=EDGE_CURVE ( 'NONE', #9500, #14160, #708, .T. ) ;
#2658=VECTOR ( 'NONE', #563, 1000.000000000000000 ) ;
#2682=ORIENTED_EDGE ( 'NONE', *, *, #17075, .F. ) ;
#2688=VERTEX_POINT ( 'NONE', #6701 ) ;
#2692=FACE_OUTER_BOUND ( 'NONE', #4779, .T. ) ;
#2696=CARTESIAN_POINT ( 'NONE',  ( -57.08002265617300708, 84.22855780814606419, -167.1454815528550739 ) ) ;
#2699=DIRECTION ( 'NONE',  ( 1.000000000000000000, 0.000000000000000000, 0.000000000000000000 ) ) ;
#2700=ORIENTED_EDGE ( 'NONE', *, *, #17709, .F. ) ;
#2707=ORIENTED_EDGE ( 'NONE', *, *, #2868, .F. ) ;
#2715=EDGE_LOOP ( 'NONE', ( #920, #6973, #18155, #7405 ) ) ;
#2716=VECTOR ( 'NONE', #9067, 1000.000000000000000 ) ;
#2733=CARTESIAN_POINT ( 'NONE',  ( -65.17806329749801364, 93.75072866207683830, -15.00000000000001243 ) ) ;
#2735=ORIENTED_EDGE ( 'NONE', *, *, #13485, .F. ) ;
#2741=ORIENTED_EDGE ( 'NONE', *, *, #297, .F. ) ;
#2742=AXIS2_PLACEMENT_3D ( 'NONE', #1450, #7153, #12870 ) ;
#2743=AXIS2_PLACEMENT_3D ( 'NONE', #13147, #4441, #5857 ) ;
#2748=CIRCLE ( 'NONE', #944, 4.599999999999999645 ) ;
#2751=DIRECTION ( 'NONE',  ( 0.000000000000000000, 0.000000000000000000, 1.000000000000000000 ) ) ;
#2767=LINE ( 'NONE', #6788, #15308 ) ;
#2773=ADVANCED_FACE ( 'NONE', ( #15695, #319 ), #5922, .T. ) ;
#2776=VECTOR ( 'NONE', #1220, 1000.000000000000000 ) ;
#2781=CARTESIAN_POINT ( 'NONE',  ( -48.74405704658271077, 91.10542963993684396, -167.1454815528550739 ) ) ;
#2791=VERTEX_POINT ( 'NONE', #17889 ) ;
#2796=CYLINDRICAL_SURFACE ( 'NONE', #967, 12.50000000000000355 ) ;
#2802=CARTESIAN_POINT ( 'NONE',  ( -47.02742034342072941, 91.65790412808885890, -167.1454815528550739 ) ) ;
#2807=CIRCLE ( 'NONE', #10544, 12.50000000000000355 ) ;
#2831=AXIS2_PLACEMENT_3D ( 'NONE', #1623, #11550, #5904 ) ;
#2836=CARTESIAN_POINT ( 'NONE',  ( -57.99147934508202695, 74.02016676429184372, -15.00000000000001421 ) ) ;
#2837=VERTEX_POINT ( 'NONE', #9397 ) ;
#2844=ORIENTED_EDGE ( 'NONE', *, *, #3221, .F. ) ;
#2849=ORIENTED_EDGE ( 'NONE', *, *, #10335, .F. ) ;
#2851=FACE_OUTER_BOUND ( 'NONE', #16830, .T. ) ;
#2855=VERTEX_POINT ( 'NONE', #18281 ) ;
#2862=DIRECTION ( 'NONE',  ( -1.000000000000000000, -6.661338147750943976E-15, 1.387778780781446662E-16 ) ) ;
#2868=EDGE_CURVE ( 'NONE', #9420, #10261, #5487, .T. ) ;
#2875=DIRECTION ( 'NONE',  ( 1.000000000000000000, 0.000000000000000000, 0.000000000000000000 ) ) ;
#2880=CARTESIAN_POINT ( 'NONE',  ( -57.08002265617300708, 84.22855780814606419, -15.00000000000001421 ) ) ;
#2884=VERTEX_POINT ( 'NONE', #18098 ) ;
#2889=VERTEX_POINT ( 'NONE', #5352 ) ;
#2894=DIRECTION ( 'NONE',  ( 1.000000000000000000, 0.000000000000000000, 0.000000000000000000 ) ) ;
#2905=ORIENTED_EDGE ( 'NONE', *, *, #9161, .T. ) ;
#2909=CARTESIAN_POINT ( 'NONE',  ( -57.08002265617300708, 84.22855780814606419, -167.1454815528550739 ) ) ;
#2922=DIRECTION ( 'NONE',  ( 0.000000000000000000, 0.000000000000000000, 1.000000000000000000 ) ) ;
#2929=VERTEX_POINT ( 'NONE', #10895 ) ;
#2940=DIRECTION ( 'NONE',  ( -1.000000000000000000, 2.109423746787799005E-14, 1.387778780781446662E-16 ) ) ;
#2951=CIRCLE ( 'NONE', #18501, 12.49999999999999645 ) ;
#2957=DIRECTION ( 'NONE',  ( -5.204170427930409450E-16, 0.000000000000000000, 1.000000000000000000 ) ) ;
#2960=DIRECTION ( 'NONE',  ( 1.156482317317869999E-16, 0.000000000000000000, 1.000000000000000000 ) ) ;
#2962=ADVANCED_FACE ( 'NONE', ( #2851 ), #4338, .T. ) ;
#2964=VECTOR ( 'NONE', #13241, 1000.000000000000000 ) ;
#2975=CIRCLE ( 'NONE', #7743, 10.24900000000000766 ) ;
#2977=VECTOR ( 'NONE', #18123, 1000.000000000000000 ) ;
#2988=DIRECTION ( 'NONE',  ( 1.000000000000000000, 0.000000000000000000, 5.077734830647302671E-16 ) ) ;
#3002=EDGE_CURVE ( 'NONE', #274, #1187, #11776, .T. ) ;
#3014=DIRECTION ( 'NONE',  ( 0.000000000000000000, 0.000000000000000000, 1.000000000000000000 ) ) ;
#3027=ORIENTED_EDGE ( 'NONE', *, *, #15319, .T. ) ;
#3028=AXIS2_PLACEMENT_3D ( 'NONE', #10906, #8283, #15184 ) ;
#3029=EDGE_LOOP ( 'NONE', ( #17481, #3932, #17533, #5533 ) ) ;
#3031=CARTESIAN_POINT ( 'NONE',  ( -57.08002265617300708, 84.22855780814606419, -15.00000000000001421 ) ) ;
#3042=CIRCLE ( 'NONE', #56, 4.600000000000006750 ) ;
#3046=DIRECTION ( 'NONE',  ( 0.000000000000000000, 0.000000000000000000, 1.000000000000000000 ) ) ;
#3047=DIRECTION ( 'NONE',  ( 1.000000000000000000, 0.000000000000000000, 3.771137991253923150E-16 ) ) ;
#3048=CYLINDRICAL_SURFACE ( 'NONE', #7497, 4.599999999999992539 ) ;
#3052=DIRECTION ( 'NONE',  ( 0.000000000000000000, 0.000000000000000000, 1.000000000000000000 ) ) ;
#3053=CARTESIAN_POINT ( 'NONE',  ( -48.65098454476478196, 77.46608744949921288, -167.1454815528550739 ) ) ;
#3068=FACE_OUTER_BOUND ( 'NONE', #7042, .T. ) ;
#3073=FACE_OUTER_BOUND ( 'NONE', #37, .T. ) ;
#3074=DIRECTION ( 'NONE',  ( 0.000000000000000000, 0.000000000000000000, 1.000000000000000000 ) ) ;
#3079=EDGE_CURVE ( 'NONE', #11670, #17138, #17736, .T. ) ;
#3080=DIRECTION ( 'NONE',  ( 1.000000000000000000, 0.000000000000000000, 5.551115123125786646E-16 ) ) ;
#3085=CARTESIAN_POINT ( 'NONE',  ( -53.44817431141344599, 74.64462966772957486, -15.00000000000001421 ) ) ;
#3087=VECTOR ( 'NONE', #256, 1000.000000000000000 ) ;
#3103=EDGE_CURVE ( 'NONE', #1000, #16773, #9006, .T. ) ;
#3115=AXIS2_PLACEMENT_3D ( 'NONE', #16141, #445, #6315 ) ;
#3116=ADVANCED_FACE ( 'NONE', ( #7870 ), #1985, .T. ) ;
#3117=AXIS2_PLACEMENT_3D ( 'NONE', #11158, #11055, #13674 ) ;
#3125=EDGE_LOOP ( 'NONE', ( #53, #5669, #3865, #17124, #6168, #17356, #13435, #10412, #14241, #477, #15134, #9001, #3749, #17717, #15653, #1934, #9819, #6511, #8617, #1701, #5467, #493, #13429, #2220, #5267, #6264, #4443, #1265, #18015, #5748, #12975, #9004, #4502, #14300, #13408, #17515, #15615, #9986, #12555, #7195, #8751, #10596, #1400, #14999, #6564, #4438, #12956, #15571, #17226, #9617, #15147, #7025, #13213, #1311, #11706, #17809, #13812, #781, #13997, #17054, #15429, #1586, #12151, #10761, #4672, #13203, #17, #8565, #9427, #6617, #10419, #14798, #2741, #18206, #10732, #13861, #14836, #18360, #17168, #519, #7980, #17026, #11221, #6130, #17141, #5619, #8711, #1993, #16461, #11597, #6014, #5345, #16094, #12015, #11041 ) ) ;
#3128=DIRECTION ( 'NONE',  ( 1.156482317317869999E-16, 0.000000000000000000, 1.000000000000000000 ) ) ;
#3145=ORIENTED_EDGE ( 'NONE', *, *, #1525, .T. ) ;
#3146=DIRECTION ( 'NONE',  ( 0.000000000000000000, 0.000000000000000000, 1.000000000000000000 ) ) ;
#3149=DIRECTION ( 'NONE',  ( -5.204170427930409450E-16, 0.000000000000000000, 1.000000000000000000 ) ) ;
#3150=VERTEX_POINT ( 'NONE', #4873 ) ;
#3151=DIRECTION ( 'NONE',  ( 0.000000000000000000, 0.000000000000000000, 1.000000000000000000 ) ) ;
#3152=CARTESIAN_POINT ( 'NONE',  ( -44.78895386838529902, 81.95267818613812949, -15.00000000000001421 ) ) ;
#3153=DIRECTION ( 'NONE',  ( -1.000000000000000000, 0.000000000000000000, 0.000000000000000000 ) ) ;
#3157=AXIS2_PLACEMENT_3D ( 'NONE', #3719, #2604, #3611 ) ;
#3174=ORIENTED_EDGE ( 'NONE', *, *, #17928, .T. ) ;
#3176=DIRECTION ( 'NONE',  ( -1.000000000000000000, 0.000000000000000000, 1.692578276882434470E-16 ) ) ;
#3177=ORIENTED_EDGE ( 'NONE', *, *, #6287, .T. ) ;
#3180=ADVANCED_FACE ( 'NONE', ( #12179 ), #14968, .T. ) ;
#3181=DIRECTION ( 'NONE',  ( -1.000000000000000000, 0.000000000000000000, 1.692578276882436442E-16 ) ) ;
#3196=EDGE_CURVE ( 'NONE', #2889, #11833, #4600, .T. ) ;
#3203=VERTEX_POINT ( 'NONE', #12666 ) ;
#3221=EDGE_CURVE ( 'NONE', #13519, #4088, #2513, .T. ) ;
#3222=DIRECTION ( 'NONE',  ( 1.000000000000000000, 0.000000000000000000, 0.000000000000000000 ) ) ;
#3238=ORIENTED_EDGE ( 'NONE', *, *, #7535, .T. ) ;
#3241=DIRECTION ( 'NONE',  ( 0.000000000000000000, 0.000000000000000000, 1.000000000000000000 ) ) ;
#3248=CARTESIAN_POINT ( 'NONE',  ( -57.56709772515574031, 94.46597735006069740, 15.00000000000006928 ) ) ;
#3250=DIRECTION ( 'NONE',  ( 1.000000000000000000, 0.000000000000000000, 3.771137991253928573E-16 ) ) ;
#3252=EDGE_LOOP ( 'NONE', ( #210, #4323, #1274, #11764 ) ) ;
#3256=VECTOR ( 'NONE', #10033, 1000.000000000000000 ) ;
#3257=ORIENTED_EDGE ( 'NONE', *, *, #4797, .F. ) ;
#3266=CARTESIAN_POINT ( 'NONE',  ( -57.08002265617300708, 84.22855780814606419, -167.1454815528550739 ) ) ;
#3269=CIRCLE ( 'NONE', #8654, 12.50000000000001066 ) ;
#3271=CARTESIAN_POINT ( 'NONE',  ( -53.44817431141344599, 74.64462966772957486, 15.00000000000006928 ) ) ;
#3276=DIRECTION ( 'NONE',  ( -1.000000000000000000, 3.016910393003138520E-15, 0.000000000000000000 ) ) ;
#3291=ORIENTED_EDGE ( 'NONE', *, *, #6289, .T. ) ;
#3299=VERTEX_POINT ( 'NONE', #18163 ) ;
#3300=EDGE_CURVE ( 'NONE', #10126, #7359, #8795, .T. ) ;
#3303=CYLINDRICAL_SURFACE ( 'NONE', #1002, 10.24900000000000055 ) ;
#3306=CARTESIAN_POINT ( 'NONE',  ( -57.08002265617300708, 84.22855780814606419, 15.00000000000006928 ) ) ;
#3307=FACE_OUTER_BOUND ( 'NONE', #7939, .T. ) ;
#3312=EDGE_CURVE ( 'NONE', #3784, #10391, #11535, .T. ) ;
#3314=DIRECTION ( 'NONE',  ( -5.204170427930409450E-16, 0.000000000000000000, 1.000000000000000000 ) ) ;
#3316=CIRCLE ( 'NONE', #10806, 12.50000000000000355 ) ;
#3323=EDGE_LOOP ( 'NONE', ( #15480, #10089, #14610, #12467 ) ) ;
#3325=EDGE_CURVE ( 'NONE', #15057, #5292, #15540, .T. ) ;
#3328=CIRCLE ( 'NONE', #17970, 10.24900000000001477 ) ;
#3329=LINE ( 'NONE', #12139, #9120 ) ;
#3330=LINE ( 'NONE', #348, #13531 ) ;
#3337=DIRECTION ( 'NONE',  ( -1.000000000000000000, -1.332267629550188795E-14, 1.387778780781446662E-16 ) ) ;
#3340=ORIENTED_EDGE ( 'NONE', *, *, #6518, .T. ) ;
#3349=AXIS2_PLACEMENT_3D ( 'NONE', #14966, #10866, #10591 ) ;
#3351=ORIENTED_EDGE ( 'NONE', *, *, #3221, .T. ) ;
#3358=FACE_OUTER_BOUND ( 'NONE', #13694, .T. ) ;
#3362=AXIS2_PLACEMENT_3D ( 'NONE', #1060, #6752, #1424 ) ;
#3364=AXIS2_PLACEMENT_3D ( 'NONE', #4721, #13171, #14565 ) ;
#3367=CARTESIAN_POINT ( 'NONE',  ( -57.08002265617300708, 84.22855780814606419, -15.00000000000001421 ) ) ;
#3369=ORIENTED_EDGE ( 'NONE', *, *, #10127, .T. ) ;
#3381=FACE_OUTER_BOUND ( 'NONE', #528, .T. ) ;
#3382=CARTESIAN_POINT ( 'NONE',  ( -63.91856434051376823, 76.59466308582156557, 15.00000000000006928 ) ) ;
#3388=AXIS2_PLACEMENT_3D ( 'NONE', #10448, #17744, #4554 ) ;
#3390=AXIS2_PLACEMENT_3D ( 'NONE', #6309, #522, #9501 ) ;
#3401=AXIS2_PLACEMENT_3D ( 'NONE', #10322, #16016, #8910 ) ;
#3403=CARTESIAN_POINT ( 'NONE',  ( -53.29103256796045684, 73.45256821284057480, 15.00000000000007105 ) ) ;
#3406=VERTEX_POINT ( 'NONE', #8440 ) ;
#3407=FACE_OUTER_BOUND ( 'NONE', #14814, .T. ) ;
#3412=AXIS2_PLACEMENT_3D ( 'NONE', #10913, #5088, #10807 ) ;
#3416=AXIS2_PLACEMENT_3D ( 'NONE', #16162, #9444, #17662 ) ;
#3417=EDGE_LOOP ( 'NONE', ( #7450, #3027, #10285, #13477 ) ) ;
#3422=CARTESIAN_POINT ( 'NONE',  ( -50.99714023269321217, 75.97988867778809663, -15.00000000000001421 ) ) ;
#3424=ORIENTED_EDGE ( 'NONE', *, *, #3552, .T. ) ;
#3427=SHAPE_REPRESENTATION_RELATIONSHIP ( 'NONE' , 'NONE' ,  #15047, #2318 ) ;
#3442=EDGE_CURVE ( 'NONE', #14366, #2307, #6217, .T. ) ;
#3446=EDGE_CURVE ( 'NONE', #16773, #8753, #5338, .T. ) ;
#3452=AXIS2_PLACEMENT_3D ( 'NONE', #8102, #13822, #1199 ) ;
#3454=DIRECTION ( 'NONE',  ( 1.156482317317869999E-16, 0.000000000000000000, 1.000000000000000000 ) ) ;
#3457=DIRECTION ( 'NONE',  ( 1.000000000000000000, 0.000000000000000000, 5.077734830647302671E-16 ) ) ;
#3459=EDGE_CURVE ( 'NONE', #11848, #583, #1870, .T. ) ;
#3460=CARTESIAN_POINT ( 'NONE',  ( -48.43547250063686960, 78.72276507608465579, -167.1454815528550739 ) ) ;
#3473=UNCERTAINTY_MEASURE_WITH_UNIT (LENGTH_MEASURE( 1.000000000000000082E-05 ), #2021, 'distance_accuracy_value', 'NONE');
#3474=DIRECTION ( 'NONE',  ( -5.204170427930409450E-16, 0.000000000000000000, 1.000000000000000000 ) ) ;
#3476=DIRECTION ( 'NONE',  ( 0.000000000000000000, 0.000000000000000000, 1.000000000000000000 ) ) ;
#3493=ADVANCED_FACE ( 'NONE', ( #17484 ), #13293, .T. ) ;
#3494=LINE ( 'NONE', #6385, #17763 ) ;
#3496=ORIENTED_EDGE ( 'NONE', *, *, #6981, .F. ) ;
#3503=CARTESIAN_POINT ( 'NONE',  ( -57.08002265617300708, 84.22855780814606419, 15.00000000000006928 ) ) ;
#3509=CARTESIAN_POINT ( 'NONE',  ( -57.08002265617300708, 84.22855780814606419, -15.00000000000001421 ) ) ;
#3511=ORIENTED_EDGE ( 'NONE', *, *, #4383, .T. ) ;
#3515=DIRECTION ( 'NONE',  ( 0.000000000000000000, 0.000000000000000000, 1.000000000000000000 ) ) ;
#3521=LINE ( 'NONE', #4833, #18304 ) ;
#3534=EDGE_CURVE ( 'NONE', #12444, #12214, #813, .T. ) ;
#3539=LINE ( 'NONE', #3460, #6696 ) ;
#3552=EDGE_CURVE ( 'NONE', #16418, #10691, #12536, .T. ) ;
#3573=EDGE_LOOP ( 'NONE', ( #10498, #11283, #13309, #15054 ) ) ;
#3582=DIRECTION ( 'NONE',  ( 0.000000000000000000, 0.000000000000000000, 1.000000000000000000 ) ) ;
#3583=DIRECTION ( 'NONE',  ( -1.000000000000000000, 0.000000000000000000, 0.000000000000000000 ) ) ;
#3586=CIRCLE ( 'NONE', #15857, 4.600000000000006750 ) ;
#3588=AXIS2_PLACEMENT_3D ( 'NONE', #13020, #4737, #13100 ) ;
#3592=AXIS2_PLACEMENT_3D ( 'NONE', #11782, #4738, #3176 ) ;
#3596=VERTEX_POINT ( 'NONE', #1386 ) ;
#3600=DIRECTION ( 'NONE',  ( 1.156482317317869999E-16, 0.000000000000000000, 1.000000000000000000 ) ) ;
#3601=VERTEX_POINT ( 'NONE', #8395 ) ;
#3606=CARTESIAN_POINT ( 'NONE',  ( -57.08002265617300708, 84.22855780814606419, -167.1454815528550739 ) ) ;
#3611=DIRECTION ( 'NONE',  ( 1.000000000000000000, 0.000000000000000000, 3.771137991253923150E-16 ) ) ;
#3624=ORIENTED_EDGE ( 'NONE', *, *, #14967, .F. ) ;
#3635=DIRECTION ( 'NONE',  ( 1.000000000000000000, 0.000000000000000000, 0.000000000000000000 ) ) ;
#3637=AXIS2_PLACEMENT_3D ( 'NONE', #18225, #1301, #5584 ) ;
#3644=DIRECTION ( 'NONE',  ( -1.000000000000000000, -2.978937767313084233E-14, 1.692578276882434470E-16 ) ) ;
#3645=CIRCLE ( 'NONE', #7537, 10.24900000000001477 ) ;
#3648=EDGE_CURVE ( 'NONE', #10547, #2688, #3849, .T. ) ;
#3649=EDGE_LOOP ( 'NONE', ( #9182, #9488, #18317, #11993 ) ) ;
#3651=AXIS2_PLACEMENT_3D ( 'NONE', #11076, #8365, #6679 ) ;
#3652=EDGE_CURVE ( 'NONE', #5943, #10611, #9705, .T. ) ;
#3653=CARTESIAN_POINT ( 'NONE',  ( -57.08002265617300708, 84.22855780814606419, 15.00000000000006928 ) ) ;
#3654=CARTESIAN_POINT ( 'NONE',  ( -57.08002265617300708, 84.22855780814606419, -15.00000000000001421 ) ) ;
#3659=VERTEX_POINT ( 'NONE', #12889 ) ;
#3665=VERTEX_POINT ( 'NONE', #6994 ) ;
#3667=DIRECTION ( 'NONE',  ( 0.000000000000000000, 0.000000000000000000, 1.000000000000000000 ) ) ;
#3676=EDGE_CURVE ( 'NONE', #13750, #7723, #7361, .T. ) ;
#3686=DIRECTION ( 'NONE',  ( 1.000000000000000000, 0.000000000000000000, 0.000000000000000000 ) ) ;
#3687=CIRCLE ( 'NONE', #14161, 10.24900000000000055 ) ;
#3689=EDGE_CURVE ( 'NONE', #9250, #12214, #15812, .T. ) ;
#3708=CIRCLE ( 'NONE', #13274, 4.599999999999992539 ) ;
#3716=CARTESIAN_POINT ( 'NONE',  ( -57.08002265617300708, 84.22855780814606419, -167.1454815528550739 ) ) ;
#3717=ORIENTED_EDGE ( 'NONE', *, *, #2652, .F. ) ;
#3719=CARTESIAN_POINT ( 'NONE',  ( -63.25151023250651150, 93.09943318379590949, 15.00000000000006928 ) ) ;
#3723=VECTOR ( 'NONE', #12338, 1000.000000000000000 ) ;
#3734=CYLINDRICAL_SURFACE ( 'NONE', #15327, 12.50000000000000355 ) ;
#3738=AXIS2_PLACEMENT_3D ( 'NONE', #12252, #13747, #6735 ) ;
#3739=CARTESIAN_POINT ( 'NONE',  ( -57.08002265617300708, 84.22855780814606419, 15.00000000000006928 ) ) ;
#3742=CARTESIAN_POINT ( 'NONE',  ( -47.02742034342072941, 91.65790412808885890, 15.00000000000009592 ) ) ;
#3749=ORIENTED_EDGE ( 'NONE', *, *, #6518, .F. ) ;
#3751=CARTESIAN_POINT ( 'NONE',  ( -57.08002265617300708, 84.22855780814606419, -167.1454815528550739 ) ) ;
#3754=EDGE_LOOP ( 'NONE', ( #17655, #17248, #10397, #16961 ) ) ;
#3755=CARTESIAN_POINT ( 'NONE',  ( -47.27059076829218043, 81.25920652595885940, 15.00000000000009592 ) ) ;
#3757=CARTESIAN_POINT ( 'NONE',  ( -57.08002265617300708, 84.22855780814606419, 15.00000000000006928 ) ) ;
#3767=CARTESIAN_POINT ( 'NONE',  ( -52.35105328106566702, 95.79950628479642205, -15.00000000000001421 ) ) ;
#3768=ORIENTED_EDGE ( 'NONE', *, *, #12268, .F. ) ;
#3769=DIRECTION ( 'NONE',  ( 0.000000000000000000, 0.000000000000000000, 1.000000000000000000 ) ) ;
#3774=DIRECTION ( 'NONE',  ( 0.000000000000000000, 0.000000000000000000, 1.000000000000000000 ) ) ;
#3782=DIRECTION ( 'NONE',  ( 1.156482317317869999E-16, 0.000000000000000000, 1.000000000000000000 ) ) ;
#3784=VERTEX_POINT ( 'NONE', #4706 ) ;
#3786=LINE ( 'NONE', #985, #16178 ) ;
#3791=EDGE_CURVE ( 'NONE', #9544, #9457, #2975, .T. ) ;
#3797=ORIENTED_EDGE ( 'NONE', *, *, #13513, .T. ) ;
#3803=LINE ( 'NONE', #6600, #575 ) ;
#3805=DIRECTION ( 'NONE',  ( 1.156482317317869999E-16, 0.000000000000000000, 1.000000000000000000 ) ) ;
#3826=DIRECTION ( 'NONE',  ( 1.000000000000000000, 0.000000000000000000, 0.000000000000000000 ) ) ;
#3832=CARTESIAN_POINT ( 'NONE',  ( -67.13262496892538422, 91.65790412808873100, -15.00000000000001421 ) ) ;
#3835=CARTESIAN_POINT ( 'NONE',  ( -47.80867013224673912, 89.78028827820993740, -15.00000000000001421 ) ) ;
#3836=ORIENTED_EDGE ( 'NONE', *, *, #7665, .F. ) ;
#3838=VERTEX_POINT ( 'NONE', #14369 ) ;
#3841=CARTESIAN_POINT ( 'NONE',  ( -60.31105839772099841, 93.95493478196522119, -167.1454815528550739 ) ) ;
#3848=ORIENTED_EDGE ( 'NONE', *, *, #11899, .T. ) ;
#3849=CIRCLE ( 'NONE', #17006, 10.24899999999998812 ) ;
#3857=ORIENTED_EDGE ( 'NONE', *, *, #3459, .F. ) ;
#3865=ORIENTED_EDGE ( 'NONE', *, *, #17928, .F. ) ;
#3875=DIRECTION ( 'NONE',  ( -1.000000000000000000, -1.218656359355351063E-14, 1.692578276882432005E-16 ) ) ;
#3876=CARTESIAN_POINT ( 'NONE',  ( -57.08002265617300708, 84.22855780814606419, 15.00000000000006928 ) ) ;
#3878=EDGE_CURVE ( 'NONE', #9354, #14934, #13422, .T. ) ;
#3879=EDGE_CURVE ( 'NONE', #14168, #15468, #4180, .T. ) ;
#3880=DIRECTION ( 'NONE',  ( 0.000000000000000000, 0.000000000000000000, 1.000000000000000000 ) ) ;
#3889=CARTESIAN_POINT ( 'NONE',  ( -53.39175999306721110, 74.07097899412303832, 15.00000000000006928 ) ) ;
#3892=LINE ( 'NONE', #624, #9966 ) ;
#3897=CARTESIAN_POINT ( 'NONE',  ( -46.36441787118067026, 82.83016482797245317, 15.00000000000009592 ) ) ;
#3902=ORIENTED_EDGE ( 'NONE', *, *, #10802, .T. ) ;
#3927=LINE ( 'NONE', #2246, #15558 ) ;
#3929=AXIS2_PLACEMENT_3D ( 'NONE', #14428, #7317, #9763 ) ;
#3932=ORIENTED_EDGE ( 'NONE', *, *, #6255, .T. ) ;
#3934=CIRCLE ( 'NONE', #14396, 10.24900000000000055 ) ;
#3935=AXIS2_PLACEMENT_3D ( 'NONE', #9084, #2050, #3635 ) ;
#3944=APPLICATION_CONTEXT ( 'automotive_design' ) ;
#3956=EDGE_CURVE ( 'NONE', #17138, #4389, #18218, .T. ) ;
#3965=CARTESIAN_POINT ( 'NONE',  ( -45.85876501399108207, 78.72098330317804482, 15.00000000000006928 ) ) ;
#3969=CARTESIAN_POINT ( 'NONE',  ( -46.89970808030100358, 83.04399200740388665, 15.00000000000006928 ) ) ;
#3974=VERTEX_POINT ( 'NONE', #5365 ) ;
#3981=CIRCLE ( 'NONE', #13844, 4.600000000000006750 ) ;
#3983=DIRECTION ( 'NONE',  ( 1.000000000000000000, 0.000000000000000000, 0.000000000000000000 ) ) ;
#3992=CARTESIAN_POINT ( 'NONE',  ( -57.08002265617300708, 84.22855780814606419, -15.00000000000001421 ) ) ;
#4000=DIRECTION ( 'NONE',  ( 1.156482317317869999E-16, 0.000000000000000000, 1.000000000000000000 ) ) ;
#4007=CYLINDRICAL_SURFACE ( 'NONE', #5386, 4.599999999999992539 ) ;
#4014=ORIENTED_EDGE ( 'NONE', *, *, #4376, .F. ) ;
#4026=AXIS2_PLACEMENT_3D ( 'NONE', #4095, #1294, #12719 ) ;
#4029=CYLINDRICAL_SURFACE ( 'NONE', #17467, 12.49999999999999645 ) ;
#4031=DIRECTION ( 'NONE',  ( 0.000000000000000000, 0.000000000000000000, 1.000000000000000000 ) ) ;
#4035=CARTESIAN_POINT ( 'NONE',  ( -52.55467279550843784, 75.03273214436886462, -15.00000000000001421 ) ) ;
#4044=CIRCLE ( 'NONE', #15075, 4.599999999999992539 ) ;
#4048=EDGE_CURVE ( 'NONE', #2327, #7640, #8956, .T. ) ;
#4054=CARTESIAN_POINT ( 'NONE',  ( -49.26569365422058411, 90.86016871721223254, -15.00000000000001421 ) ) ;
#4057=ORIENTED_EDGE ( 'NONE', *, *, #5828, .F. ) ;
#4062=AXIS2_PLACEMENT_3D ( 'NONE', #18224, #16806, #15311 ) ;
#4086=ADVANCED_FACE ( 'NONE', ( #11730 ), #17421, .T. ) ;
#4088=VERTEX_POINT ( 'NONE', #13061 ) ;
#4094=DIRECTION ( 'NONE',  ( -1.000000000000000000, 0.000000000000000000, 0.000000000000000000 ) ) ;
#4095=CARTESIAN_POINT ( 'NONE',  ( -57.08002265617300708, 84.22855780814606419, 15.00000000000006928 ) ) ;
#4098=CARTESIAN_POINT ( 'NONE',  ( -53.44605150580733266, 72.26844686893191749, -15.00000000000001421 ) ) ;
#4101=DIRECTION ( 'NONE',  ( 1.000000000000000000, 0.000000000000000000, 0.000000000000000000 ) ) ;
#4102=EDGE_LOOP ( 'NONE', ( #511, #3424, #18298, #7956 ) ) ;
#4105=DIRECTION ( 'NONE',  ( 0.000000000000000000, 0.000000000000000000, 1.000000000000000000 ) ) ;
#4113=LINE ( 'NONE', #15518, #692 ) ;
#4117=CYLINDRICAL_SURFACE ( 'NONE', #8541, 10.24900000000000055 ) ;
#4118=CARTESIAN_POINT ( 'NONE',  ( -62.81538793034061285, 92.72253132893551708, -15.00000000000001421 ) ) ;
#4120=ORIENTED_EDGE ( 'NONE', *, *, #10135, .T. ) ;
#4121=EDGE_CURVE ( 'NONE', #2855, #3150, #3269, .T. ) ;
#4128=ORIENTED_EDGE ( 'NONE', *, *, #17270, .T. ) ;
#4141=ORIENTED_EDGE ( 'NONE', *, *, #7780, .T. ) ;
#4142=CARTESIAN_POINT ( 'NONE',  ( -57.08002265617300708, 84.22855780814606419, -15.00000000000001421 ) ) ;
#4151=ORIENTED_EDGE ( 'NONE', *, *, #8674, .F. ) ;
#4166=CARTESIAN_POINT ( 'NONE',  ( -47.13906347517657025, 79.99098546104539764, -15.00000000000001421 ) ) ;
#4173=CARTESIAN_POINT ( 'NONE',  ( -59.20641439073742873, 73.63336328296978195, -167.1454815528550739 ) ) ;
#4180=CIRCLE ( 'NONE', #5349, 10.24900000000001477 ) ;
#4195=EDGE_LOOP ( 'NONE', ( #4991, #10816, #5222, #6077 ) ) ;
#4198=DIRECTION ( 'NONE',  ( -5.204170427930409450E-16, 0.000000000000000000, 1.000000000000000000 ) ) ;
#4200=VERTEX_POINT ( 'NONE', #14617 ) ;
#4203=DIRECTION ( 'NONE',  ( 1.000000000000000000, 0.000000000000000000, 5.204170427930409450E-16 ) ) ;
#4205=AXIS2_PLACEMENT_3D ( 'NONE', #4399, #15895, #16940 ) ;
#4212=AXIS2_PLACEMENT_3D ( 'NONE', #4652, #15977, #352 ) ;
#4219=VERTEX_POINT ( 'NONE', #782 ) ;
#4227=FACE_OUTER_BOUND ( 'NONE', #5264, .T. ) ;
#4230=ORIENTED_EDGE ( 'NONE', *, *, #5620, .F. ) ;
#4232=EDGE_CURVE ( 'NONE', #11248, #7349, #2371, .T. ) ;
#4236=AXIS2_PLACEMENT_3D ( 'NONE', #15652, #14333, #17303 ) ;
#4253=DIRECTION ( 'NONE',  ( 1.000000000000000000, 0.000000000000000000, 3.771137991253934490E-16 ) ) ;
#4262=VERTEX_POINT ( 'NONE', #3767 ) ;
#4263=CARTESIAN_POINT ( 'NONE',  ( -67.02098183716937285, 79.99098546104525553, -15.00000000000001421 ) ) ;
#4267=ORIENTED_EDGE ( 'NONE', *, *, #16258, .T. ) ;
#4293=CARTESIAN_POINT ( 'NONE',  ( -57.08002265617300708, 84.22855780814606419, 15.00000000000006928 ) ) ;
#4294=ORIENTED_EDGE ( 'NONE', *, *, #12082, .T. ) ;
#4297=DIRECTION ( 'NONE',  ( 1.000000000000000000, 0.000000000000000000, 5.077734830647299712E-16 ) ) ;
#4314=AXIS2_PLACEMENT_3D ( 'NONE', #2781, #9700, #2875 ) ;
#4323=ORIENTED_EDGE ( 'NONE', *, *, #1601, .T. ) ;
#4333=AXIS2_PLACEMENT_3D ( 'NONE', #16070, #13106, #3181 ) ;
#4335=EDGE_CURVE ( 'NONE', #14981, #2271, #12484, .T. ) ;
#4337=EDGE_CURVE ( 'NONE', #4498, #4736, #11169, .T. ) ;
#4338=CYLINDRICAL_SURFACE ( 'NONE', #2831, 12.50000000000000355 ) ;
#4349=ORIENTED_EDGE ( 'NONE', *, *, #7237, .F. ) ;
#4357=CIRCLE ( 'NONE', #15992, 4.599999999999999645 ) ;
#4360=EDGE_CURVE ( 'NONE', #14903, #848, #11054, .T. ) ;
#4376=EDGE_CURVE ( 'NONE', #8935, #9204, #7, .T. ) ;
#4377=DIRECTION ( 'NONE',  ( 1.000000000000000000, 0.000000000000000000, 3.771137991253928573E-16 ) ) ;
#4379=LINE ( 'NONE', #15964, #6282 ) ;
#4380=CARTESIAN_POINT ( 'NONE',  ( -45.21333244822126574, 88.15687341518456321, -15.00000000000001421 ) ) ;
#4383=EDGE_CURVE ( 'NONE', #15468, #4644, #6244, .T. ) ;
#4389=VERTEX_POINT ( 'NONE', #1695 ) ;
#4391=DIRECTION ( 'NONE',  ( 1.156482317317869999E-16, 0.000000000000000000, 1.000000000000000000 ) ) ;
#4399=CARTESIAN_POINT ( 'NONE',  ( -57.89103256796045116, 73.45256821284057480, -15.00000000000001421 ) ) ;
#4401=ORIENTED_EDGE ( 'NONE', *, *, #1290, .F. ) ;
#4412=CARTESIAN_POINT ( 'NONE',  ( -44.89980253466632831, 81.41924511788819530, -167.1454815528550739 ) ) ;
#4414=CARTESIAN_POINT ( 'NONE',  ( -59.37303238940180705, 94.21775734381046163, 15.00000000000006928 ) ) ;
#4431=ORIENTED_EDGE ( 'NONE', *, *, #9865, .F. ) ;
#4433=ORIENTED_EDGE ( 'NONE', *, *, #16777, .T. ) ;
#4438=ORIENTED_EDGE ( 'NONE', *, *, #7306, .F. ) ;
#4441=DIRECTION ( 'NONE',  ( 0.000000000000000000, 0.000000000000000000, 1.000000000000000000 ) ) ;
#4443=ORIENTED_EDGE ( 'NONE', *, *, #14538, .F. ) ;
#4444=CARTESIAN_POINT ( 'NONE',  ( -57.08002265617300708, 84.22855780814606419, -15.00000000000001421 ) ) ;
#4448=ORIENTED_EDGE ( 'NONE', *, *, #8615, .T. ) ;
#4452=EDGE_CURVE ( 'NONE', #6195, #11833, #1610, .T. ) ;
#4456=EDGE_CURVE ( 'NONE', #2929, #8972, #14354, .T. ) ;
#4461=AXIS2_PLACEMENT_3D ( 'NONE', #6842, #2557, #7132 ) ;
#4463=CARTESIAN_POINT ( 'NONE',  ( -49.75809927370887920, 76.28065702765852052, -15.00000000000001421 ) ) ;
#4465=PLANE ( 'NONE',  #11487 ) ;
#4470=DIRECTION ( 'NONE',  ( -5.204170427930409450E-16, 0.000000000000000000, 1.000000000000000000 ) ) ;
#4473=EDGE_CURVE ( 'NONE', #10126, #14988, #15746, .T. ) ;
#4474=EDGE_CURVE ( 'NONE', #15130, #13519, #11974, .T. ) ;
#4476=AXIS2_PLACEMENT_3D ( 'NONE', #7321, #17043, #14159 ) ;
#4477=ORIENTED_EDGE ( 'NONE', *, *, #10156, .F. ) ;
#4480=VECTOR ( 'NONE', #5577, 1000.000000000000000 ) ;
#4481=DIRECTION ( 'NONE',  ( 1.000000000000000000, 0.000000000000000000, 5.077734830647295768E-16 ) ) ;
#4493=AXIS2_PLACEMENT_3D ( 'NONE', #13454, #13552, #8019 ) ;
#4498=VERTEX_POINT ( 'NONE', #14781 ) ;
#4501=CARTESIAN_POINT ( 'NONE',  ( -57.08002265617300708, 84.22855780814606419, -167.1454815528550739 ) ) ;
#4502=ORIENTED_EDGE ( 'NONE', *, *, #6181, .F. ) ;
#4514=DIRECTION ( 'NONE',  ( 1.156482317317869999E-16, 0.000000000000000000, 1.000000000000000000 ) ) ;
#4517=CIRCLE ( 'NONE', #11982, 10.24900000000000055 ) ;
#4520=VERTEX_POINT ( 'NONE', #14685 ) ;
#4523=VECTOR ( 'NONE', #9659, 1000.000000000000000 ) ;
#4528=CARTESIAN_POINT ( 'NONE',  ( -50.24148097183213935, 76.59466308582166505, -167.1454815528550739 ) ) ;
#4540=DIRECTION ( 'NONE',  ( 1.000000000000000000, 0.000000000000000000, 0.000000000000000000 ) ) ;
#4554=DIRECTION ( 'NONE',  ( -1.000000000000000000, -5.551115123125786646E-15, 1.387778780781446662E-16 ) ) ;
#4557=DIRECTION ( 'NONE',  ( 1.000000000000000000, 0.000000000000000000, 0.000000000000000000 ) ) ;
#4565=ORIENTED_EDGE ( 'NONE', *, *, #9858, .T. ) ;
#4585=AXIS2_PLACEMENT_3D ( 'NONE', #12321, #2016, #5199 ) ;
#4592=ORIENTED_EDGE ( 'NONE', *, *, #7062, .T. ) ;
#4593=DIRECTION ( 'NONE',  ( -1.000000000000000000, 0.000000000000000000, 0.000000000000000000 ) ) ;
#4600=CIRCLE ( 'NONE', #12396, 4.599999999999992539 ) ;
#4602=CARTESIAN_POINT ( 'NONE',  ( -57.08002265617300708, 84.22855780814606419, 15.00000000000006928 ) ) ;
#4604=CARTESIAN_POINT ( 'NONE',  ( -57.08002265617300708, 84.22855780814606419, -15.00000000000001421 ) ) ;
#4616=VERTEX_POINT ( 'NONE', #4035 ) ;
#4617=CARTESIAN_POINT ( 'NONE',  ( -63.91856434051376823, 76.59466308582156557, -167.1454815528550739 ) ) ;
#4619=CIRCLE ( 'NONE', #18384, 4.599999999999992539 ) ;
#4621=AXIS2_PLACEMENT_3D ( 'NONE', #13252, #8949, #4540 ) ;
#4627=DIRECTION ( 'NONE',  ( -5.204170427930409450E-16, 0.000000000000000000, 1.000000000000000000 ) ) ;
#4628=DIRECTION ( 'NONE',  ( -1.000000000000000000, 0.000000000000000000, 0.000000000000000000 ) ) ;
#4632=CARTESIAN_POINT ( 'NONE',  ( -67.46561775476841660, 81.24207102880470188, 15.00000000000006928 ) ) ;
#4634=ORIENTED_EDGE ( 'NONE', *, *, #3689, .F. ) ;
#4639=FACE_OUTER_BOUND ( 'NONE', #12369, .T. ) ;
#4644=VERTEX_POINT ( 'NONE', #3832 ) ;
#4645=DIRECTION ( 'NONE',  ( -5.204170427930409450E-16, 0.000000000000000000, 1.000000000000000000 ) ) ;
#4651=ORIENTED_EDGE ( 'NONE', *, *, #2655, .F. ) ;
#4652=CARTESIAN_POINT ( 'NONE',  ( -61.98611128973170992, 74.59995546124152099, -167.1454815528550739 ) ) ;
#4660=CARTESIAN_POINT ( 'NONE',  ( -60.62932119839002354, 94.43552448259767118, 15.00000000000006928 ) ) ;
#4671=CARTESIAN_POINT ( 'NONE',  ( -44.59353464447068660, 84.80960611389554060, 15.00000000000006928 ) ) ;
#4672=ORIENTED_EDGE ( 'NONE', *, *, #16691, .F. ) ;
#4678=EDGE_CURVE ( 'NONE', #2791, #11538, #2147, .T. ) ;
#4681=ORIENTED_EDGE ( 'NONE', *, *, #15039, .F. ) ;
#4689=EDGE_CURVE ( 'NONE', #18116, #3150, #3927, .T. ) ;
#4691=CYLINDRICAL_SURFACE ( 'NONE', #332, 10.24900000000001477 ) ;
#4694=DIRECTION ( 'NONE',  ( 1.156482317317869999E-16, 0.000000000000000000, 1.000000000000000000 ) ) ;
#4698=EDGE_CURVE ( 'NONE', #4736, #9544, #5378, .T. ) ;
#4705=EDGE_LOOP ( 'NONE', ( #17288, #12237, #5225, #13510 ) ) ;
#4706=CARTESIAN_POINT ( 'NONE',  ( -59.05157857372951469, 96.57209730311865314, -15.00000000000001421 ) ) ;
#4707=CYLINDRICAL_SURFACE ( 'NONE', #2743, 4.599999999999999645 ) ;
#4715=CYLINDRICAL_SURFACE ( 'NONE', #4621, 10.24900000000000055 ) ;
#4717=CYLINDRICAL_SURFACE ( 'NONE', #15210, 4.600000000000006750 ) ;
#4721=CARTESIAN_POINT ( 'NONE',  ( -67.46561775476841660, 81.24207102880470188, -167.1454815528550739 ) ) ;
#4736=VERTEX_POINT ( 'NONE', #13853 ) ;
#4737=DIRECTION ( 'NONE',  ( -5.204170427930409450E-16, 0.000000000000000000, 1.000000000000000000 ) ) ;
#4738=DIRECTION ( 'NONE',  ( 1.156482317317869999E-16, 0.000000000000000000, 1.000000000000000000 ) ) ;
#4753=AXIS2_PLACEMENT_3D ( 'NONE', #6787, #11091, #15188 ) ;
#4762=VECTOR ( 'NONE', #11448, 1000.000000000000000 ) ;
#4765=AXIS2_PLACEMENT_3D ( 'NONE', #15733, #5700, #5794 ) ;
#4766=DIRECTION ( 'NONE',  ( -5.204170427930409450E-16, 0.000000000000000000, 1.000000000000000000 ) ) ;
#4777=AXIS2_PLACEMENT_3D ( 'NONE', #4293, #15715, #8411 ) ;
#4779=EDGE_LOOP ( 'NONE', ( #4786, #3174, #15655, #17331 ) ) ;
#4780=VECTOR ( 'NONE', #12460, 1000.000000000000000 ) ;
#4783=AXIS2_PLACEMENT_3D ( 'NONE', #6711, #7093, #15307 ) ;
#4786=ORIENTED_EDGE ( 'NONE', *, *, #14642, .F. ) ;
#4790=EDGE_LOOP ( 'NONE', ( #18408, #8428, #10519, #15677 ) ) ;
#4797=EDGE_CURVE ( 'NONE', #18335, #8753, #17291, .T. ) ;
#4802=ORIENTED_EDGE ( 'NONE', *, *, #3002, .T. ) ;
#4806=DIRECTION ( 'NONE',  ( 1.000000000000000000, 0.000000000000000000, 0.000000000000000000 ) ) ;
#4811=AXIS2_PLACEMENT_3D ( 'NONE', #17794, #1898, #14888 ) ;
#4814=EDGE_CURVE ( 'NONE', #8556, #18489, #1416, .T. ) ;
#4816=ORIENTED_EDGE ( 'NONE', *, *, #11450, .T. ) ;
#4817=ORIENTED_EDGE ( 'NONE', *, *, #10762, .T. ) ;
#4820=AXIS2_PLACEMENT_3D ( 'NONE', #169, #11653, #17264 ) ;
#4823=CARTESIAN_POINT ( 'NONE',  ( -57.08002265617300708, 84.22855780814606419, -167.1454815528550739 ) ) ;
#4825=LINE ( 'NONE', #11855, #12696 ) ;
#4827=CARTESIAN_POINT ( 'NONE',  ( -50.81952187608693805, 73.40930968350535579, -15.00000000000001421 ) ) ;
#4828=AXIS2_PLACEMENT_3D ( 'NONE', #428, #6116, #6200 ) ;
#4829=AXIS2_PLACEMENT_3D ( 'NONE', #2624, #9534, #16723 ) ;
#4831=DIRECTION ( 'NONE',  ( 1.000000000000000000, 0.000000000000000000, 0.000000000000000000 ) ) ;
#4833=CARTESIAN_POINT ( 'NONE',  ( -45.39578445746348478, 88.67024416760654049, -167.1454815528550739 ) ) ;
#4835=CARTESIAN_POINT ( 'NONE',  ( -53.97067643794850511, 72.12145385653101926, -167.1454815528550739 ) ) ;
#4840=DIRECTION ( 'NONE',  ( 0.000000000000000000, 0.000000000000000000, 1.000000000000000000 ) ) ;
#4842=ORIENTED_EDGE ( 'NONE', *, *, #6982, .T. ) ;
#4853=CARTESIAN_POINT ( 'NONE',  ( -62.81538793034061285, 92.72253132893551708, 15.00000000000006928 ) ) ;
#4860=AXIS2_PLACEMENT_3D ( 'NONE', #832, #3454, #5028 ) ;
#4864=CYLINDRICAL_SURFACE ( 'NONE', #544, 4.600000000000006750 ) ;
#4865=ORIENTED_EDGE ( 'NONE', *, *, #1831, .T. ) ;
#4873=CARTESIAN_POINT ( 'NONE',  ( -49.40461175531926585, 94.09456345901895702, 15.00000000000006928 ) ) ;
#4897=CIRCLE ( 'NONE', #1667, 12.50000000000000355 ) ;
#4899=AXIS2_PLACEMENT_3D ( 'NONE', #7476, #13196, #17482 ) ;
#4911=CIRCLE ( 'NONE', #15976, 12.50000000000001066 ) ;
#4916=ORIENTED_EDGE ( 'NONE', *, *, #466, .F. ) ;
#4924=DIRECTION ( 'NONE',  ( 0.000000000000000000, 0.000000000000000000, 1.000000000000000000 ) ) ;
#4930=FACE_OUTER_BOUND ( 'NONE', #15374, .T. ) ;
#4933=EDGE_CURVE ( 'NONE', #14988, #11134, #17927, .T. ) ;
#4964=DIRECTION ( 'NONE',  ( 1.156482317317869999E-16, 0.000000000000000000, 1.000000000000000000 ) ) ;
#4965=DIRECTION ( 'NONE',  ( -5.204170427930409450E-16, 0.000000000000000000, 1.000000000000000000 ) ) ;
#4970=VERTEX_POINT ( 'NONE', #13098 ) ;
#4971=DIRECTION ( 'NONE',  ( 0.000000000000000000, 0.000000000000000000, 1.000000000000000000 ) ) ;
#4981=EDGE_CURVE ( 'NONE', #15230, #2837, #363, .T. ) ;
#4989=EDGE_CURVE ( 'NONE', #8149, #16609, #16256, .T. ) ;
#4990=DIRECTION ( 'NONE',  ( 1.000000000000000000, 0.000000000000000000, 3.771137991253934490E-16 ) ) ;
#4991=ORIENTED_EDGE ( 'NONE', *, *, #15221, .F. ) ;
#5011=CARTESIAN_POINT ( 'NONE',  ( -67.79562744116532258, 82.83016482797231106, -167.1454815528550739 ) ) ;
#5013=DIRECTION ( 'NONE',  ( 0.000000000000000000, 0.000000000000000000, 1.000000000000000000 ) ) ;
#5023=EDGE_CURVE ( 'NONE', #2884, #703, #10764, .T. ) ;
#5028=DIRECTION ( 'NONE',  ( -1.000000000000000000, 0.000000000000000000, 0.000000000000000000 ) ) ;
#5046=EDGE_LOOP ( 'NONE', ( #4151, #5098, #16028, #15742 ) ) ;
#5050=DIRECTION ( 'NONE',  ( -1.000000000000000000, 0.000000000000000000, 0.000000000000000000 ) ) ;
#5052=AXIS2_PLACEMENT_3D ( 'NONE', #6470, #17518, #16027 ) ;
#5055=ORIENTED_EDGE ( 'NONE', *, *, #2552, .T. ) ;
#5073=DIRECTION ( 'NONE',  ( 0.000000000000000000, 0.000000000000000000, 1.000000000000000000 ) ) ;
#5075=VECTOR ( 'NONE', #12906, 1000.000000000000000 ) ;
#5076=CARTESIAN_POINT ( 'NONE',  ( -64.89435165812551531, 90.86016871721213306, 15.00000000000006928 ) ) ;
#5083=CIRCLE ( 'NONE', #3588, 4.599999999999992539 ) ;
#5084=DIRECTION ( 'NONE',  ( 1.156482317317869999E-16, 0.000000000000000000, 1.000000000000000000 ) ) ;
#5088=DIRECTION ( 'NONE',  ( -5.204170427930409450E-16, 0.000000000000000000, 1.000000000000000000 ) ) ;
#5098=ORIENTED_EDGE ( 'NONE', *, *, #16344, .T. ) ;
#5101=DIRECTION ( 'NONE',  ( 0.000000000000000000, 0.000000000000000000, 1.000000000000000000 ) ) ;
#5107=DIRECTION ( 'NONE',  ( -5.204170427930409450E-16, 0.000000000000000000, 1.000000000000000000 ) ) ;
#5116=CARTESIAN_POINT ( 'NONE',  ( -47.15582643534892782, 86.78830982163900387, 15.00000000000006928 ) ) ;
#5126=CARTESIAN_POINT ( 'NONE',  ( -67.26033723204500347, 83.04399200740374454, -15.00000000000001243 ) ) ;
#5129=DIRECTION ( 'NONE',  ( 1.000000000000000000, 0.000000000000000000, 0.000000000000000000 ) ) ;
#5139=AXIS2_PLACEMENT_3D ( 'NONE', #3654, #6548, #17967 ) ;
#5141=AXIS2_PLACEMENT_3D ( 'NONE', #12651, #4031, #6924 ) ;
#5148=ORIENTED_EDGE ( 'NONE', *, *, #15790, .F. ) ;
#5155=CIRCLE ( 'NONE', #10837, 4.600000000000006750 ) ;
#5157=CIRCLE ( 'NONE', #1299, 4.599999999999992539 ) ;
#5165=EDGE_CURVE ( 'NONE', #7640, #16893, #18229, .T. ) ;
#5188=ORIENTED_EDGE ( 'NONE', *, *, #4232, .T. ) ;
#5199=DIRECTION ( 'NONE',  ( 1.000000000000000000, 0.000000000000000000, 0.000000000000000000 ) ) ;
#5217=LINE ( 'NONE', #4835, #14193 ) ;
#5219=ORIENTED_EDGE ( 'NONE', *, *, #4121, .F. ) ;
#5222=ORIENTED_EDGE ( 'NONE', *, *, #15349, .T. ) ;
#5225=ORIENTED_EDGE ( 'NONE', *, *, #10037, .T. ) ;
#5227=AXIS2_PLACEMENT_3D ( 'NONE', #16051, #3241, #8960 ) ;
#5237=DIRECTION ( 'NONE',  ( -1.000000000000000000, -3.016910393003142859E-15, 0.000000000000000000 ) ) ;
#5243=AXIS2_PLACEMENT_3D ( 'NONE', #12624, #16521, #9511 ) ;
#5263=CARTESIAN_POINT ( 'NONE',  ( -46.71322837820016360, 91.21279551874765446, -167.1454815528550739 ) ) ;
#5264=EDGE_LOOP ( 'NONE', ( #13325, #17454, #6782, #8580 ) ) ;
#5267=ORIENTED_EDGE ( 'NONE', *, *, #815, .F. ) ;
#5270=ORIENTED_EDGE ( 'NONE', *, *, #15349, .F. ) ;
#5279=EDGE_LOOP ( 'NONE', ( #16180, #5447, #10584, #9122 ) ) ;
#5284=CYLINDRICAL_SURFACE ( 'NONE', #1280, 4.599999999999992539 ) ;
#5291=EDGE_LOOP ( 'NONE', ( #17605, #18491, #13193, #4916 ) ) ;
#5292=VERTEX_POINT ( 'NONE', #9903 ) ;
#5297=CARTESIAN_POINT ( 'NONE',  ( -65.17806329749801364, 93.75072866207683830, -167.1454815528550739 ) ) ;
#5303=DIRECTION ( 'NONE',  ( 0.000000000000000000, 0.000000000000000000, 1.000000000000000000 ) ) ;
#5315=DIRECTION ( 'NONE',  ( 0.000000000000000000, 0.000000000000000000, 1.000000000000000000 ) ) ;
#5322=DIRECTION ( 'NONE',  ( -5.204170427930409450E-16, 0.000000000000000000, 1.000000000000000000 ) ) ;
#5327=DIRECTION ( 'NONE',  ( 1.156482317317869999E-16, 0.000000000000000000, 1.000000000000000000 ) ) ;
#5338=CIRCLE ( 'NONE', #1766, 4.599999999999999645 ) ;
#5345=ORIENTED_EDGE ( 'NONE', *, *, #8614, .F. ) ;
#5349=AXIS2_PLACEMENT_3D ( 'NONE', #12699, #16681, #3875 ) ;
#5352=CARTESIAN_POINT ( 'NONE',  ( -53.44605150580733266, 72.26844686893191749, 15.00000000000006928 ) ) ;
#5361=ADVANCED_FACE ( 'NONE', ( #502 ), #17601, .T. ) ;
#5365=CARTESIAN_POINT ( 'NONE',  ( -55.10846673861666289, 96.57209730311868157, 15.00000000000006928 ) ) ;
#5366=DIRECTION ( 'NONE',  ( 1.000000000000000000, 0.000000000000000000, 3.771137991253917233E-16 ) ) ;
#5373=ORIENTED_EDGE ( 'NONE', *, *, #6981, .T. ) ;
#5378=CIRCLE ( 'NONE', #8697, 4.599999999999999645 ) ;
#5386=AXIS2_PLACEMENT_3D ( 'NONE', #16916, #4105, #12903 ) ;
#5394=FACE_OUTER_BOUND ( 'NONE', #5886, .T. ) ;
#5397=CIRCLE ( 'NONE', #3592, 10.24900000000000055 ) ;
#5409=AXIS2_PLACEMENT_3D ( 'NONE', #15576, #11469, #15758 ) ;
#5413=ORIENTED_EDGE ( 'NONE', *, *, #3312, .T. ) ;
#5417=CARTESIAN_POINT ( 'NONE',  ( -57.08002265617300708, 84.22855780814606419, -167.1454815528550739 ) ) ;
#5429=EDGE_LOOP ( 'NONE', ( #2312, #14083, #16242, #3768 ) ) ;
#5443=DIRECTION ( 'NONE',  ( 0.000000000000000000, 0.000000000000000000, 1.000000000000000000 ) ) ;
#5447=ORIENTED_EDGE ( 'NONE', *, *, #11701, .T. ) ;
#5455=DIRECTION ( 'NONE',  ( 1.000000000000000000, 0.000000000000000000, 5.551115123125784674E-16 ) ) ;
#5456=CARTESIAN_POINT ( 'NONE',  ( -57.08002265617300708, 84.22855780814606419, -167.1454815528550739 ) ) ;
#5462=EDGE_LOOP ( 'NONE', ( #16423, #5593, #16168, #2411 ) ) ;
#5464=LINE ( 'NONE', #12305, #11402 ) ;
#5467=ORIENTED_EDGE ( 'NONE', *, *, #18072, .F. ) ;
#5469=CARTESIAN_POINT ( 'NONE',  ( -65.50906076758114693, 77.46608744949911340, 15.00000000000006928 ) ) ;
#5477=ORIENTED_EDGE ( 'NONE', *, *, #1381, .F. ) ;
#5479=DIRECTION ( 'NONE',  ( 0.000000000000000000, 0.000000000000000000, 1.000000000000000000 ) ) ;
#5482=EDGE_LOOP ( 'NONE', ( #6474, #8602, #2206, #12134 ) ) ;
#5485=LINE ( 'NONE', #11108, #2977 ) ;
#5487=CIRCLE ( 'NONE', #15942, 12.49999999999999645 ) ;
#5494=FACE_OUTER_BOUND ( 'NONE', #6611, .T. ) ;
#5499=DIRECTION ( 'NONE',  ( 1.000000000000000000, 0.000000000000000000, 0.000000000000000000 ) ) ;
#5529=AXIS2_PLACEMENT_3D ( 'NONE', #4602, #10129, #14694 ) ;
#5533=ORIENTED_EDGE ( 'NONE', *, *, #7750, .F. ) ;
#5542=AXIS2_PLACEMENT_3D ( 'NONE', #3367, #9091, #3644 ) ;
#5551=ORIENTED_EDGE ( 'NONE', *, *, #18201, .F. ) ;
#5556=ORIENTED_EDGE ( 'NONE', *, *, #6058, .T. ) ;
#5559=CARTESIAN_POINT ( 'NONE',  ( -49.58002265617300708, 84.22855780814606419, -167.1454815528550739 ) ) ;
#5561=CARTESIAN_POINT ( 'NONE',  ( -54.78701292294434211, 94.21775734381050427, -167.1454815528550739 ) ) ;
#5567=VERTEX_POINT ( 'NONE', #2569 ) ;
#5577=DIRECTION ( 'NONE',  ( 0.000000000000000000, 0.000000000000000000, 1.000000000000000000 ) ) ;
#5578=DIRECTION ( 'NONE',  ( 1.156482317317869999E-16, 0.000000000000000000, 1.000000000000000000 ) ) ;
#5582=CARTESIAN_POINT ( 'NONE',  ( -67.20241558018224737, 85.83453492254335515, 15.00000000000006928 ) ) ;
#5584=DIRECTION ( 'NONE',  ( 1.000000000000000000, 0.000000000000000000, 3.771137991253928573E-16 ) ) ;
#5586=EDGE_LOOP ( 'NONE', ( #15005, #1794, #12689, #17874 ) ) ;
#5593=ORIENTED_EDGE ( 'NONE', *, *, #13977, .T. ) ;
#5595=ADVANCED_FACE ( 'NONE', ( #18092 ), #18275, .T. ) ;
#5598=DIRECTION ( 'NONE',  ( 0.000000000000000000, 0.000000000000000000, 1.000000000000000000 ) ) ;
#5599=LINE ( 'NONE', #8127, #12041 ) ;
#5603=CYLINDRICAL_SURFACE ( 'NONE', #15420, 4.599999999999999645 ) ;
#5606=ORIENTED_EDGE ( 'NONE', *, *, #5925, .F. ) ;
#5609=DIRECTION ( 'NONE',  ( 0.000000000000000000, 0.000000000000000000, 1.000000000000000000 ) ) ;
#5612=EDGE_CURVE ( 'NONE', #16752, #9640, #14162, .T. ) ;
#5618=ORIENTED_EDGE ( 'NONE', *, *, #4456, .T. ) ;
#5619=ORIENTED_EDGE ( 'NONE', *, *, #3079, .F. ) ;
#5620=EDGE_CURVE ( 'NONE', #7505, #9854, #1739, .T. ) ;
#5624=DIRECTION ( 'NONE',  ( -1.000000000000000000, 0.000000000000000000, 1.387778780781445182E-16 ) ) ;
#5626=EDGE_CURVE ( 'NONE', #2271, #15616, #14297, .T. ) ;
#5627=CARTESIAN_POINT ( 'NONE',  ( -56.59294758719027385, 94.46597735006069740, -167.1454815528550739 ) ) ;
#5630=CYLINDRICAL_SURFACE ( 'NONE', #11413, 4.599999999999992539 ) ;
#5639=ADVANCED_FACE ( 'NONE', ( #14259 ), #17312, .T. ) ;
#5646=ORIENTED_EDGE ( 'NONE', *, *, #12858, .F. ) ;
#5654=DIRECTION ( 'NONE',  ( -1.000000000000000000, 0.000000000000000000, 0.000000000000000000 ) ) ;
#5666=DIRECTION ( 'NONE',  ( 0.000000000000000000, 0.000000000000000000, 1.000000000000000000 ) ) ;
#5669=ORIENTED_EDGE ( 'NONE', *, *, #16915, .F. ) ;
#5674=VERTEX_POINT ( 'NONE', #4414 ) ;
#5691=DIRECTION ( 'NONE',  ( 1.000000000000000000, 0.000000000000000000, 5.551115123125780730E-16 ) ) ;
#5700=DIRECTION ( 'NONE',  ( 0.000000000000000000, 0.000000000000000000, 1.000000000000000000 ) ) ;
#5705=ORIENTED_EDGE ( 'NONE', *, *, #13085, .T. ) ;
#5712=EDGE_CURVE ( 'NONE', #9457, #1289, #9832, .T. ) ;
#5723=EDGE_CURVE ( 'NONE', #4262, #3659, #7715, .T. ) ;
#5724=VECTOR ( 'NONE', #860, 1000.000000000000000 ) ;
#5726=AXIS2_PLACEMENT_3D ( 'NONE', #7951, #840, #2143 ) ;
#5728=ORIENTED_EDGE ( 'NONE', *, *, #15103, .F. ) ;
#5730=EDGE_CURVE ( 'NONE', #15130, #9307, #17575, .T. ) ;
#5748=ORIENTED_EDGE ( 'NONE', *, *, #17130, .F. ) ;
#5749=ADVANCED_FACE ( 'NONE', ( #1980 ), #4864, .T. ) ;
#5755=DIRECTION ( 'NONE',  ( 1.000000000000000000, 0.000000000000000000, 0.000000000000000000 ) ) ;
#5756=CARTESIAN_POINT ( 'NONE',  ( -47.76628296033400289, 88.50596986196467242, -15.00000000000001421 ) ) ;
#5776=VERTEX_POINT ( 'NONE', #17499 ) ;
#5780=CARTESIAN_POINT ( 'NONE',  ( -67.02098183716937285, 79.99098546104525553, -167.1454815528550739 ) ) ;
#5781=CARTESIAN_POINT ( 'NONE',  ( 0.000000000000000000, 0.000000000000000000, 0.000000000000000000 ) ) ;
#5789=DIRECTION ( 'NONE',  ( -5.204170427930409450E-16, 0.000000000000000000, 1.000000000000000000 ) ) ;
#5790=CIRCLE ( 'NONE', #14183, 4.600000000000013856 ) ;
#5794=DIRECTION ( 'NONE',  ( 1.000000000000000000, 0.000000000000000000, 0.000000000000000000 ) ) ;
#5797=EDGE_LOOP ( 'NONE', ( #15037, #1414, #11077, #13591 ) ) ;
#5808=CYLINDRICAL_SURFACE ( 'NONE', #4236, 10.24899999999998812 ) ;
#5813=DIRECTION ( 'NONE',  ( 1.156482317317869999E-16, 0.000000000000000000, 1.000000000000000000 ) ) ;
#5817=AXIS2_PLACEMENT_3D ( 'NONE', #7484, #475, #2940 ) ;
#5828=EDGE_CURVE ( 'NONE', #7123, #1024, #6453, .T. ) ;
#5831=CIRCLE ( 'NONE', #5845, 4.599999999999992539 ) ;
#5832=AXIS2_PLACEMENT_3D ( 'NONE', #4823, #16239, #17542 ) ;
#5836=CARTESIAN_POINT ( 'NONE',  ( -56.16856596726385220, 74.02016676429185793, -15.00000000000001421 ) ) ;
#5837=DIRECTION ( 'NONE',  ( -1.000000000000000000, 0.000000000000000000, 0.000000000000000000 ) ) ;
#5845=AXIS2_PLACEMENT_3D ( 'NONE', #6133, #14839, #17548 ) ;
#5846=CIRCLE ( 'NONE', #16292, 10.24900000000000055 ) ;
#5852=EDGE_CURVE ( 'NONE', #7640, #15247, #9220, .T. ) ;
#5857=DIRECTION ( 'NONE',  ( 1.000000000000000000, 0.000000000000000000, 0.000000000000000000 ) ) ;
#5866=EDGE_CURVE ( 'NONE', #18116, #3203, #8023, .T. ) ;
#5875=CARTESIAN_POINT ( 'NONE',  ( -65.72457281170906640, 78.72276507608454210, -167.1454815528550739 ) ) ;
#5878=EDGE_LOOP ( 'NONE', ( #369, #15220, #5705, #2844 ) ) ;
#5882=CARTESIAN_POINT ( 'NONE',  ( -47.15582643534892782, 86.78830982163900387, -15.00000000000001421 ) ) ;
#5886=EDGE_LOOP ( 'NONE', ( #17028, #11122, #6024, #17250 ) ) ;
#5894=DIRECTION ( 'NONE',  ( 1.000000000000000000, 0.000000000000000000, 3.771137991253934490E-16 ) ) ;
#5899=CARTESIAN_POINT ( 'NONE',  ( -46.83322972390671879, 84.01587117655466841, -15.00000000000001421 ) ) ;
#5903=DIRECTION ( 'NONE',  ( 1.000000000000000000, 0.000000000000000000, 0.000000000000000000 ) ) ;
#5904=DIRECTION ( 'NONE',  ( 1.000000000000000000, 0.000000000000000000, 0.000000000000000000 ) ) ;
#5912=ADVANCED_FACE ( 'NONE', ( #15150 ), #13952, .T. ) ;
#5922=PLANE ( 'NONE',  #1604 ) ;
#5925=EDGE_CURVE ( 'NONE', #17041, #7723, #2951, .T. ) ;
#5936=CARTESIAN_POINT ( 'NONE',  ( -57.74389692835771370, 95.01461175692088545, -15.00000000000001421 ) ) ;
#5941=DIRECTION ( 'NONE',  ( 0.000000000000000000, 0.000000000000000000, 1.000000000000000000 ) ) ;
#5943=VERTEX_POINT ( 'NONE', #3085 ) ;
#5953=ORIENTED_EDGE ( 'NONE', *, *, #8507, .F. ) ;
#5956=EDGE_CURVE ( 'NONE', #14934, #3601, #8332, .T. ) ;
#5957=DIRECTION ( 'NONE',  ( 1.000000000000000000, 0.000000000000000000, 0.000000000000000000 ) ) ;
#5962=VECTOR ( 'NONE', #13476, 1000.000000000000000 ) ;
#5968=EDGE_LOOP ( 'NONE', ( #10878, #15428, #1152, #16507 ) ) ;
#5973=CARTESIAN_POINT ( 'NONE',  ( -64.50972932340006594, 92.07579602767982863, -15.00000000000001421 ) ) ;
#5977=AXIS2_PLACEMENT_3D ( 'NONE', #4660, #17653, #10458 ) ;
#5986=VECTOR ( 'NONE', #10001, 1000.000000000000000 ) ;
#5993=ORIENTED_EDGE ( 'NONE', *, *, #4981, .F. ) ;
#5997=DIRECTION ( 'NONE',  ( 1.156482317317869999E-16, 0.000000000000000000, 1.000000000000000000 ) ) ;
#6008=AXIS2_PLACEMENT_3D ( 'NONE', #859, #9377, #15076 ) ;
#6009=ORIENTED_EDGE ( 'NONE', *, *, #1497, .F. ) ;
#6014=ORIENTED_EDGE ( 'NONE', *, *, #4360, .F. ) ;
#6015=CARTESIAN_POINT ( 'NONE',  ( -64.50972932340006594, 92.07579602767982863, 15.00000000000006928 ) ) ;
#6021=DIRECTION ( 'NONE',  ( 1.000000000000000000, 0.000000000000000000, 0.000000000000000000 ) ) ;
#6022=DIRECTION ( 'NONE',  ( 1.000000000000000000, 0.000000000000000000, 3.771137991253934490E-16 ) ) ;
#6024=ORIENTED_EDGE ( 'NONE', *, *, #13278, .T. ) ;
#6036=VECTOR ( 'NONE', #14614, 1000.000000000000000 ) ;
#6037=DIRECTION ( 'NONE',  ( 0.000000000000000000, 0.000000000000000000, 1.000000000000000000 ) ) ;
#6045=DIRECTION ( 'NONE',  ( 0.000000000000000000, 0.000000000000000000, 1.000000000000000000 ) ) ;
#6046=LINE ( 'NONE', #16147, #72 ) ;
#6048=CIRCLE ( 'NONE', #18330, 7.500000000000000000 ) ;
#6056=ORIENTED_EDGE ( 'NONE', *, *, #6283, .T. ) ;
#6058=EDGE_CURVE ( 'NONE', #17079, #17041, #11333, .T. ) ;
#6060=EDGE_CURVE ( 'NONE', #1931, #6195, #13461, .T. ) ;
#6062=CIRCLE ( 'NONE', #1014, 4.599999999999992539 ) ;
#6077=ORIENTED_EDGE ( 'NONE', *, *, #1612, .F. ) ;
#6085=CARTESIAN_POINT ( 'NONE',  ( -57.89103256796045116, 73.45256821284057480, 15.00000000000006928 ) ) ;
#6087=ORIENTED_EDGE ( 'NONE', *, *, #17595, .F. ) ;
#6091=DIRECTION ( 'NONE',  ( -1.000000000000000000, -3.016910393003138520E-15, 0.000000000000000000 ) ) ;
#6109=VERTEX_POINT ( 'NONE', #8706 ) ;
#6112=CARTESIAN_POINT ( 'NONE',  ( -56.41614838398844256, 95.01461175692088545, -15.00000000000001421 ) ) ;
#6116=DIRECTION ( 'NONE',  ( 0.000000000000000000, 0.000000000000000000, 1.000000000000000000 ) ) ;
#6118=ORIENTED_EDGE ( 'NONE', *, *, #10335, .T. ) ;
#6120=FACE_OUTER_BOUND ( 'NONE', #6307, .T. ) ;
#6129=LINE ( 'NONE', #13441, #12984 ) ;
#6130=ORIENTED_EDGE ( 'NONE', *, *, #12728, .F. ) ;
#6133=CARTESIAN_POINT ( 'NONE',  ( -67.79562744116532258, 82.83016482797231106, -15.00000000000001421 ) ) ;
#6135=DIRECTION ( 'NONE',  ( 1.000000000000000000, 0.000000000000000000, 3.771137991253934490E-16 ) ) ;
#6140=CARTESIAN_POINT ( 'NONE',  ( -49.93060289285580922, 91.57211267264388255, -167.1454815528550739 ) ) ;
#6155=EDGE_LOOP ( 'NONE', ( #7487, #3511, #15396, #4014 ) ) ;
#6165=EDGE_CURVE ( 'NONE', #15625, #8437, #17558, .T. ) ;
#6168=ORIENTED_EDGE ( 'NONE', *, *, #3002, .F. ) ;
#6169=EDGE_CURVE ( 'NONE', #4644, #9204, #2038, .T. ) ;
#6181=EDGE_CURVE ( 'NONE', #3203, #2791, #1799, .T. ) ;
#6186=ORIENTED_EDGE ( 'NONE', *, *, #2283, .T. ) ;
#6189=ORIENTED_EDGE ( 'NONE', *, *, #12899, .F. ) ;
#6195=VERTEX_POINT ( 'NONE', #16064 ) ;
#6196=EDGE_CURVE ( 'NONE', #8556, #1000, #5397, .T. ) ;
#6200=DIRECTION ( 'NONE',  ( 1.000000000000000000, 0.000000000000000000, 0.000000000000000000 ) ) ;
#6217=CIRCLE ( 'NONE', #14896, 4.599999999999999645 ) ;
#6218=CARTESIAN_POINT ( 'NONE',  ( -55.10846673861666289, 96.57209730311868157, -167.1454815528550739 ) ) ;
#6226=ORIENTED_EDGE ( 'NONE', *, *, #8510, .T. ) ;
#6231=ORIENTED_EDGE ( 'NONE', *, *, #311, .F. ) ;
#6244=CIRCLE ( 'NONE', #16119, 4.600000000000006750 ) ;
#6255=EDGE_CURVE ( 'NONE', #11356, #1931, #8405, .T. ) ;
#6259=CIRCLE ( 'NONE', #5977, 4.599999999999999645 ) ;
#6260=DIRECTION ( 'NONE',  ( 0.000000000000000000, 0.000000000000000000, 1.000000000000000000 ) ) ;
#6264=ORIENTED_EDGE ( 'NONE', *, *, #11684, .F. ) ;
#6270=DIRECTION ( 'NONE',  ( 1.000000000000000000, 0.000000000000000000, 0.000000000000000000 ) ) ;
#6276=VECTOR ( 'NONE', #5609, 1000.000000000000000 ) ;
#6278=VERTEX_POINT ( 'NONE', #4380 ) ;
#6282=VECTOR ( 'NONE', #10086, 1000.000000000000000 ) ;
#6283=EDGE_CURVE ( 'NONE', #3665, #7505, #17924, .T. ) ;
#6287=EDGE_CURVE ( 'NONE', #11552, #15616, #9907, .T. ) ;
#6289=EDGE_CURVE ( 'NONE', #18359, #17247, #17195, .T. ) ;
#6291=AXIS2_PLACEMENT_3D ( 'NONE', #17618, #17530, #14723 ) ;
#6292=FACE_OUTER_BOUND ( 'NONE', #14862, .T. ) ;
#6298=DIRECTION ( 'NONE',  ( 1.000000000000000000, 0.000000000000000000, 5.077734830647295768E-16 ) ) ;
#6302=DIRECTION ( 'NONE',  ( 1.156482317317869999E-16, 0.000000000000000000, 1.000000000000000000 ) ) ;
#6304=CIRCLE ( 'NONE', #6612, 4.599999999999992539 ) ;
#6306=ORIENTED_EDGE ( 'NONE', *, *, #11684, .T. ) ;
#6307=EDGE_LOOP ( 'NONE', ( #10343, #15749, #6797, #17422 ) ) ;
#6309=CARTESIAN_POINT ( 'NONE',  ( -57.08002265617300708, 84.22855780814606419, -167.1454815528550739 ) ) ;
#6313=CARTESIAN_POINT ( 'NONE',  ( -54.80923614058017534, 94.79374675277698259, -167.1454815528550739 ) ) ;
#6315=DIRECTION ( 'NONE',  ( 1.000000000000000000, 0.000000000000000000, 0.000000000000000000 ) ) ;
#6317=CYLINDRICAL_SURFACE ( 'NONE', #10470, 4.599999999999992539 ) ;
#6321=CARTESIAN_POINT ( 'NONE',  ( -46.38449965345759551, 85.77305660501679085, -15.00000000000001421 ) ) ;
#6328=CIRCLE ( 'NONE', #13811, 4.599999999999999645 ) ;
#6329=LINE ( 'NONE', #2131, #9881 ) ;
#6332=ORIENTED_EDGE ( 'NONE', *, *, #12082, .F. ) ;
#6339=DIRECTION ( 'NONE',  ( 1.156482317317869999E-16, 0.000000000000000000, 1.000000000000000000 ) ) ;
#6371=EDGE_LOOP ( 'NONE', ( #5477, #12108, #2282, #2735 ) ) ;
#6382=ADVANCED_FACE ( 'NONE', ( #12809 ), #15786, .T. ) ;
#6385=CARTESIAN_POINT ( 'NONE',  ( -48.13268001719898592, 75.49957964911752129, -167.1454815528550739 ) ) ;
#6396=EDGE_CURVE ( 'NONE', #15625, #15720, #15249, .T. ) ;
#6404=EDGE_CURVE ( 'NONE', #10454, #13894, #9573, .T. ) ;
#6410=ADVANCED_FACE ( 'NONE', ( #10992 ), #18194, .T. ) ;
#6414=CARTESIAN_POINT ( 'NONE',  ( -47.13906347517657025, 79.99098546104539764, 15.00000000000009592 ) ) ;
#6415=CARTESIAN_POINT ( 'NONE',  ( -57.56709772515574031, 94.46597735006069740, -167.1454815528550739 ) ) ;
#6420=ORIENTED_EDGE ( 'NONE', *, *, #15221, .T. ) ;
#6427=DIRECTION ( 'NONE',  ( 1.000000000000000000, 0.000000000000000000, 0.000000000000000000 ) ) ;
#6429=EDGE_CURVE ( 'NONE', #16609, #16158, #14955, .T. ) ;
#6432=EDGE_CURVE ( 'NONE', #2011, #70, #5464, .T. ) ;
#6433=ORIENTED_EDGE ( 'NONE', *, *, #6289, .F. ) ;
#6437=ORIENTED_EDGE ( 'NONE', *, *, #4689, .F. ) ;
#6443=CARTESIAN_POINT ( 'NONE',  ( -54.75080917176597950, 94.79374675277695417, -15.00000000000001421 ) ) ;
#6450=DIRECTION ( 'NONE',  ( 0.000000000000000000, 0.000000000000000000, 1.000000000000000000 ) ) ;
#6453=LINE ( 'NONE', #13384, #2658 ) ;
#6457=DIRECTION ( 'NONE',  ( 1.156482317317869999E-16, 0.000000000000000000, 1.000000000000000000 ) ) ;
#6466=FACE_OUTER_BOUND ( 'NONE', #17781, .T. ) ;
#6470=CARTESIAN_POINT ( 'NONE',  ( -57.08002265617300708, 84.22855780814606419, 15.00000000000006928 ) ) ;
#6474=ORIENTED_EDGE ( 'NONE', *, *, #18277, .F. ) ;
#6476=FACE_OUTER_BOUND ( 'NONE', #10481, .T. ) ;
#6502=CARTESIAN_POINT ( 'NONE',  ( -61.80899203128051056, 95.79950628479635100, -167.1454815528550739 ) ) ;
#6504=DIRECTION ( 'NONE',  ( 1.000000000000000000, 0.000000000000000000, 0.000000000000000000 ) ) ;
#6505=ORIENTED_EDGE ( 'NONE', *, *, #2283, .F. ) ;
#6509=AXIS2_PLACEMENT_3D ( 'NONE', #7060, #12772, #15659 ) ;
#6511=ORIENTED_EDGE ( 'NONE', *, *, #12951, .F. ) ;
#6515=CYLINDRICAL_SURFACE ( 'NONE', #14490, 10.24900000000000766 ) ;
#6518=EDGE_CURVE ( 'NONE', #1656, #15261, #17060, .T. ) ;
#6527=EDGE_CURVE ( 'NONE', #616, #3601, #8566, .T. ) ;
#6528=CARTESIAN_POINT ( 'NONE',  ( -57.08002265617300708, 84.22855780814606419, -15.00000000000001421 ) ) ;
#6532=CYLINDRICAL_SURFACE ( 'NONE', #2387, 10.24900000000000055 ) ;
#6545=EDGE_LOOP ( 'NONE', ( #654, #10782, #3902, #15143 ) ) ;
#6547=CARTESIAN_POINT ( 'NONE',  ( -54.80923614058017534, 94.79374675277698259, 15.00000000000006928 ) ) ;
#6548=DIRECTION ( 'NONE',  ( 1.156482317317869999E-16, 0.000000000000000000, 1.000000000000000000 ) ) ;
#6552=DIRECTION ( 'NONE',  ( 0.000000000000000000, 0.000000000000000000, 1.000000000000000000 ) ) ;
#6553=CIRCLE ( 'NONE', #16403, 10.24900000000000055 ) ;
#6558=CARTESIAN_POINT ( 'NONE',  ( -60.71399380653853228, 72.26844686893187486, 15.00000000000006928 ) ) ;
#6563=DIRECTION ( 'NONE',  ( 0.000000000000000000, 0.000000000000000000, 1.000000000000000000 ) ) ;
#6564=ORIENTED_EDGE ( 'NONE', *, *, #539, .F. ) ;
#6593=AXIS2_PLACEMENT_3D ( 'NONE', #14084, #2583, #12306 ) ;
#6594=AXIS2_PLACEMENT_3D ( 'NONE', #13076, #4627, #13333 ) ;
#6597=CARTESIAN_POINT ( 'NONE',  ( -48.74405704658271077, 91.10542963993684396, -15.00000000000001421 ) ) ;
#6600=CARTESIAN_POINT ( 'NONE',  ( -67.20241558018224737, 85.83453492254335515, -167.1454815528550739 ) ) ;
#6611=EDGE_LOOP ( 'NONE', ( #18113, #3340, #9771, #15323 ) ) ;
#6612=AXIS2_PLACEMENT_3D ( 'NONE', #1856, #14498, #6135 ) ;
#6616=EDGE_CURVE ( 'NONE', #9284, #2271, #6913, .T. ) ;
#6617=ORIENTED_EDGE ( 'NONE', *, *, #1025, .F. ) ;
#6630=CARTESIAN_POINT ( 'NONE',  ( -62.81538793034061285, 92.72253132893551708, -167.1454815528550739 ) ) ;
#6633=DIRECTION ( 'NONE',  ( 0.000000000000000000, 0.000000000000000000, 1.000000000000000000 ) ) ;
#6639=DIRECTION ( 'NONE',  ( -1.000000000000000000, 0.000000000000000000, 0.000000000000000000 ) ) ;
#6651=ORIENTED_EDGE ( 'NONE', *, *, #1042, .F. ) ;
#6663=LINE ( 'NONE', #13593, #4523 ) ;
#6679=DIRECTION ( 'NONE',  ( 1.000000000000000000, 0.000000000000000000, 5.551115123125786646E-16 ) ) ;
#6680=ORIENTED_EDGE ( 'NONE', *, *, #1612, .T. ) ;
#6690=DIRECTION ( 'NONE',  ( -1.000000000000000000, 0.000000000000000000, 0.000000000000000000 ) ) ;
#6696=VECTOR ( 'NONE', #17485, 1000.000000000000000 ) ;
#6698=AXIS2_PLACEMENT_3D ( 'NONE', #4604, #14528, #8642 ) ;
#6701=CARTESIAN_POINT ( 'NONE',  ( -60.71187100093244737, 74.64462966772953223, -15.00000000000001421 ) ) ;
#6707=FACE_OUTER_BOUND ( 'NONE', #5046, .T. ) ;
#6708=ORIENTED_EDGE ( 'NONE', *, *, #7357, .T. ) ;
#6711=CARTESIAN_POINT ( 'NONE',  ( -53.53072411395612562, 94.43552448259771381, -167.1454815528550739 ) ) ;
#6718=AXIS2_PLACEMENT_3D ( 'NONE', #7265, #18498, #16800 ) ;
#6727=AXIS2_PLACEMENT_3D ( 'NONE', #10392, #14869, #17311 ) ;
#6730=AXIS2_PLACEMENT_3D ( 'NONE', #5780, #8783, #11511 ) ;
#6735=DIRECTION ( 'NONE',  ( 1.000000000000000000, 0.000000000000000000, 0.000000000000000000 ) ) ;
#6736=DIRECTION ( 'NONE',  ( 0.000000000000000000, 0.000000000000000000, 1.000000000000000000 ) ) ;
#6741=VERTEX_POINT ( 'NONE', #579 ) ;
#6744=AXIS2_PLACEMENT_3D ( 'NONE', #9234, #630, #4831 ) ;
#6745=DIRECTION ( 'NONE',  ( 1.000000000000000000, 0.000000000000000000, 0.000000000000000000 ) ) ;
#6746=AXIS2_PLACEMENT_3D ( 'NONE', #13012, #187, #1946 ) ;
#6747=EDGE_LOOP ( 'NONE', ( #1282, #3145, #8482, #14268 ) ) ;
#6752=DIRECTION ( 'NONE',  ( 1.156482317317869999E-16, 0.000000000000000000, 1.000000000000000000 ) ) ;
#6753=ADVANCED_FACE ( 'NONE', ( #3381 ), #4691, .T. ) ;
#6782=ORIENTED_EDGE ( 'NONE', *, *, #2041, .T. ) ;
#6786=ORIENTED_EDGE ( 'NONE', *, *, #14303, .F. ) ;
#6787=CARTESIAN_POINT ( 'NONE',  ( -49.65031598894605480, 92.07579602767992810, 15.00000000000006928 ) ) ;
#6788=CARTESIAN_POINT ( 'NONE',  ( -52.55467279550843784, 75.03273214436886462, -167.1454815528550739 ) ) ;
#6792=ORIENTED_EDGE ( 'NONE', *, *, #13278, .F. ) ;
#6797=ORIENTED_EDGE ( 'NONE', *, *, #12858, .T. ) ;
#6806=CYLINDRICAL_SURFACE ( 'NONE', #14124, 4.599999999999999645 ) ;
#6808=ORIENTED_EDGE ( 'NONE', *, *, #6181, .T. ) ;
#6814=EDGE_CURVE ( 'NONE', #7359, #8149, #10209, .T. ) ;
#6816=FACE_OUTER_BOUND ( 'NONE', #2715, .T. ) ;
#6823=EDGE_LOOP ( 'NONE', ( #1139, #1643, #1542, #8140 ) ) ;
#6827=ORIENTED_EDGE ( 'NONE', *, *, #3878, .F. ) ;
#6829=CARTESIAN_POINT ( 'NONE',  ( -52.17699016282484337, 93.22868410554724505, -167.1454815528550739 ) ) ;
#6842=CARTESIAN_POINT ( 'NONE',  ( -46.27380910617147691, 84.15481808402802244, -15.00000000000001421 ) ) ;
#6843=CARTESIAN_POINT ( 'NONE',  ( -60.31105839772099841, 93.95493478196522119, 15.00000000000006928 ) ) ;
#6869=LINE ( 'NONE', #10054, #1353 ) ;
#6883=ORIENTED_EDGE ( 'NONE', *, *, #10741, .T. ) ;
#6885=EDGE_CURVE ( 'NONE', #6195, #5943, #10490, .T. ) ;
#6886=ORIENTED_EDGE ( 'NONE', *, *, #13513, .F. ) ;
#6889=EDGE_CURVE ( 'NONE', #15247, #2633, #6663, .T. ) ;
#6890=ORIENTED_EDGE ( 'NONE', *, *, #12118, .F. ) ;
#6904=DIRECTION ( 'NONE',  ( 0.000000000000000000, 0.000000000000000000, 1.000000000000000000 ) ) ;
#6913=CIRCLE ( 'NONE', #8998, 4.599999999999999645 ) ;
#6920=AXIS2_PLACEMENT_3D ( 'NONE', #15863, #3052, #6021 ) ;
#6924=DIRECTION ( 'NONE',  ( 1.000000000000000000, 0.000000000000000000, 0.000000000000000000 ) ) ;
#6937=VERTEX_POINT ( 'NONE', #9556 ) ;
#6947=CARTESIAN_POINT ( 'NONE',  ( -51.85133027979232878, 95.58244595420329404, -15.00000000000001421 ) ) ;
#6953=ORIENTED_EDGE ( 'NONE', *, *, #717, .F. ) ;
#6959=AXIS2_PLACEMENT_3D ( 'NONE', #3876, #12600, #15584 ) ;
#6967=DIRECTION ( 'NONE',  ( -5.204170427930409450E-16, 0.000000000000000000, 1.000000000000000000 ) ) ;
#6973=ORIENTED_EDGE ( 'NONE', *, *, #2178, .T. ) ;
#6981=EDGE_CURVE ( 'NONE', #3596, #14710, #7504, .T. ) ;
#6982=EDGE_CURVE ( 'NONE', #9400, #1024, #3316, .T. ) ;
#6985=CIRCLE ( 'NONE', #15335, 10.24900000000001477 ) ;
#6994=CARTESIAN_POINT ( 'NONE',  ( -48.13268001719898592, 75.49957964911752129, 15.00000000000006928 ) ) ;
#6999=VERTEX_POINT ( 'NONE', #1607 ) ;
#7009=ADVANCED_FACE ( 'NONE', ( #14335 ), #5630, .T. ) ;
#7014=EDGE_CURVE ( 'NONE', #7349, #1231, #16469, .T. ) ;
#7016=VERTEX_POINT ( 'NONE', #6947 ) ;
#7025=ORIENTED_EDGE ( 'NONE', *, *, #12616, .F. ) ;
#7030=EDGE_CURVE ( 'NONE', #848, #10424, #11708, .T. ) ;
#7032=AXIS2_PLACEMENT_3D ( 'NONE', #6528, #10841, #12245 ) ;
#7033=LINE ( 'NONE', #9449, #2776 ) ;
#7041=VERTEX_POINT ( 'NONE', #12767 ) ;
#7042=EDGE_LOOP ( 'NONE', ( #17814, #1254, #11492, #8289 ) ) ;
#7044=AXIS2_PLACEMENT_3D ( 'NONE', #3266, #17568, #14948 ) ;
#7045=AXIS2_PLACEMENT_3D ( 'NONE', #9144, #17742, #1937 ) ;
#7046=ORIENTED_EDGE ( 'NONE', *, *, #9865, .T. ) ;
#7056=CARTESIAN_POINT ( 'NONE',  ( -45.85876501399108207, 78.72098330317804482, -167.1454815528550739 ) ) ;
#7060=CARTESIAN_POINT ( 'NONE',  ( -57.08002265617300708, 84.22855780814606419, 15.00000000000006928 ) ) ;
#7062=EDGE_CURVE ( 'NONE', #10261, #16893, #17360, .T. ) ;
#7071=EDGE_LOOP ( 'NONE', ( #4477, #13671, #8282, #9085 ) ) ;
#7078=ORIENTED_EDGE ( 'NONE', *, *, #9858, .F. ) ;
#7089=DIRECTION ( 'NONE',  ( -1.000000000000000000, 2.220446049250314659E-15, 1.387778780781446662E-16 ) ) ;
#7093=DIRECTION ( 'NONE',  ( 0.000000000000000000, 0.000000000000000000, 1.000000000000000000 ) ) ;
#7105=CARTESIAN_POINT ( 'NONE',  ( -57.08002265617300708, 84.22855780814606419, 15.00000000000006928 ) ) ;
#7111=ADVANCED_FACE ( 'NONE', ( #13204 ), #17397, .T. ) ;
#7113=EDGE_CURVE ( 'NONE', #3601, #17247, #2748, .T. ) ;
#7123=VERTEX_POINT ( 'NONE', #13300 ) ;
#7129=CARTESIAN_POINT ( 'NONE',  ( -59.20641439073742873, 73.63336328296978195, -15.00000000000001421 ) ) ;
#7130=DIRECTION ( 'NONE',  ( 1.000000000000000000, 0.000000000000000000, 3.771137991253928573E-16 ) ) ;
#7132=DIRECTION ( 'NONE',  ( -1.000000000000000000, 6.033820786006295184E-15, 0.000000000000000000 ) ) ;
#7133=CARTESIAN_POINT ( 'NONE',  ( -52.35105328106566702, 95.79950628479642205, 15.00000000000006928 ) ) ;
#7145=AXIS2_PLACEMENT_3D ( 'NONE', #14690, #12173, #3276 ) ;
#7153=DIRECTION ( 'NONE',  ( 0.000000000000000000, 0.000000000000000000, 1.000000000000000000 ) ) ;
#7161=VECTOR ( 'NONE', #5941, 1000.000000000000000 ) ;
#7163=CYLINDRICAL_SURFACE ( 'NONE', #14746, 12.50000000000000355 ) ;
#7164=CARTESIAN_POINT ( 'NONE',  ( -127.5926225674731995, 47.87487112387803023, -15.00000000000000355 ) ) ;
#7170=CARTESIAN_POINT ( 'NONE',  ( -57.08002265617300708, 84.22855780814606419, -15.00000000000001421 ) ) ;
#7182=DIRECTION ( 'NONE',  ( 1.156482317317869999E-16, 0.000000000000000000, 1.000000000000000000 ) ) ;
#7184=ORIENTED_EDGE ( 'NONE', *, *, #16915, .T. ) ;
#7188=CIRCLE ( 'NONE', #17619, 12.50000000000001066 ) ;
#7189=CARTESIAN_POINT ( 'NONE',  ( -64.58002265617299997, 84.22855780814606419, -167.1454815528550739 ) ) ;
#7195=ORIENTED_EDGE ( 'NONE', *, *, #1601, .F. ) ;
#7198=DIRECTION ( 'NONE',  ( -1.000000000000000000, 1.218656359355352799E-14, 1.692578276882434470E-16 ) ) ;
#7202=AXIS2_PLACEMENT_3D ( 'NONE', #11777, #17472, #10455 ) ;
#7215=AXIS2_PLACEMENT_3D ( 'NONE', #9485, #9871, #18108 ) ;
#7224=CARTESIAN_POINT ( 'NONE',  ( -56.41614838398844256, 95.01461175692088545, -167.1454815528550739 ) ) ;
#7227=CARTESIAN_POINT ( 'NONE',  ( -61.60537251683745552, 75.03273214436880778, -15.00000000000001421 ) ) ;
#7228=ADVANCED_FACE ( 'NONE', ( #5394 ), #6806, .T. ) ;
#7230=DIRECTION ( 'NONE',  ( 0.000000000000000000, 0.000000000000000000, 1.000000000000000000 ) ) ;
#7232=AXIS2_PLACEMENT_3D ( 'NONE', #12567, #2452, #9660 ) ;
#7234=DIRECTION ( 'NONE',  ( 1.000000000000000000, 0.000000000000000000, 0.000000000000000000 ) ) ;
#7237=EDGE_CURVE ( 'NONE', #538, #14988, #7530, .T. ) ;
#7239=DIRECTION ( 'NONE',  ( 1.000000000000000000, 0.000000000000000000, 3.771137991253928573E-16 ) ) ;
#7244=AXIS2_PLACEMENT_3D ( 'NONE', #15982, #8882, #14575 ) ;
#7249=LINE ( 'NONE', #17514, #6036 ) ;
#7255=AXIS2_PLACEMENT_3D ( 'NONE', #7788, #2171, #2266 ) ;
#7262=CARTESIAN_POINT ( 'NONE',  ( -46.71322837820016360, 91.21279551874765446, -15.00000000000001421 ) ) ;
#7265=CARTESIAN_POINT ( 'NONE',  ( -57.08002265617300708, 84.22855780814606419, 15.00000000000006928 ) ) ;
#7267=CARTESIAN_POINT ( 'NONE',  ( -57.35243698450333483, 71.73152654333280509, 15.00000000000006928 ) ) ;
#7269=CIRCLE ( 'NONE', #1590, 4.599999999999999645 ) ;
#7270=AXIS2_PLACEMENT_3D ( 'NONE', #7105, #4198, #4297 ) ;
#7280=ORIENTED_EDGE ( 'NONE', *, *, #5023, .T. ) ;
#7292=FACE_OUTER_BOUND ( 'NONE', #4790, .T. ) ;
#7301=DIRECTION ( 'NONE',  ( -5.204170427930409450E-16, 0.000000000000000000, 1.000000000000000000 ) ) ;
#7306=EDGE_CURVE ( 'NONE', #7123, #1636, #16171, .T. ) ;
#7309=AXIS2_PLACEMENT_3D ( 'NONE', #17388, #11699, #201 ) ;
#7317=DIRECTION ( 'NONE',  ( -5.204170427930409450E-16, 0.000000000000000000, 1.000000000000000000 ) ) ;
#7318=ORIENTED_EDGE ( 'NONE', *, *, #12240, .T. ) ;
#7321=CARTESIAN_POINT ( 'NONE',  ( -67.77554565888843285, 85.77305660501664875, -15.00000000000001421 ) ) ;
#7325=CARTESIAN_POINT ( 'NONE',  ( -52.17393402261416213, 74.59995546124159205, 15.00000000000006928 ) ) ;
#7338=CIRCLE ( 'NONE', #6746, 10.24900000000000055 ) ;
#7343=DIRECTION ( 'NONE',  ( 1.156482317317869999E-16, 0.000000000000000000, 1.000000000000000000 ) ) ;
#7349=VERTEX_POINT ( 'NONE', #11578 ) ;
#7350=ADVANCED_FACE ( 'NONE', ( #14375 ), #328, .T. ) ;
#7355=EDGE_CURVE ( 'NONE', #17247, #3974, #12926, .T. ) ;
#7357=EDGE_CURVE ( 'NONE', #16195, #2018, #958, .T. ) ;
#7359=VERTEX_POINT ( 'NONE', #3152 ) ;
#7360=LINE ( 'NONE', #12797, #11638 ) ;
#7361=LINE ( 'NONE', #11489, #2964 ) ;
#7373=CYLINDRICAL_SURFACE ( 'NONE', #2485, 4.599999999999992539 ) ;
#7376=DIRECTION ( 'NONE',  ( 0.000000000000000000, 0.000000000000000000, 1.000000000000000000 ) ) ;
#7378=FACE_OUTER_BOUND ( 'NONE', #8658, .T. ) ;
#7379=DIRECTION ( 'NONE',  ( -5.204170427930409450E-16, 0.000000000000000000, 1.000000000000000000 ) ) ;
#7386=DIRECTION ( 'NONE',  ( 1.000000000000000000, 0.000000000000000000, 0.000000000000000000 ) ) ;
#7394=DIRECTION ( 'NONE',  ( -5.204170427930409450E-16, 0.000000000000000000, 1.000000000000000000 ) ) ;
#7405=ORIENTED_EDGE ( 'NONE', *, *, #1727, .F. ) ;
#7415=CARTESIAN_POINT ( 'NONE',  ( -55.20348911625212907, 74.15281352429526862, -15.00000000000001421 ) ) ;
#7424=ORIENTED_EDGE ( 'NONE', *, *, #12727, .T. ) ;
#7431=CARTESIAN_POINT ( 'NONE',  ( -48.65098454476478196, 77.46608744949921288, 15.00000000000006928 ) ) ;
#7438=AXIS2_PLACEMENT_3D ( 'NONE', #6015, #8938, #3047 ) ;
#7439=ADVANCED_FACE ( 'NONE', ( #3407 ), #17812, .T. ) ;
#7441=CARTESIAN_POINT ( 'NONE',  ( -57.08002265617300708, 84.22855780814606419, 15.00000000000006928 ) ) ;
#7443=EDGE_CURVE ( 'NONE', #4219, #2450, #9322, .T. ) ;
#7446=FACE_OUTER_BOUND ( 'NONE', #12810, .T. ) ;
#7450=ORIENTED_EDGE ( 'NONE', *, *, #17243, .F. ) ;
#7454=VECTOR ( 'NONE', #14055, 1000.000000000000000 ) ;
#7457=DIRECTION ( 'NONE',  ( 0.000000000000000000, 0.000000000000000000, 1.000000000000000000 ) ) ;
#7462=DIRECTION ( 'NONE',  ( -1.000000000000000000, 0.000000000000000000, 0.000000000000000000 ) ) ;
#7476=CARTESIAN_POINT ( 'NONE',  ( -57.08002265617300708, 84.22855780814606419, 15.00000000000006928 ) ) ;
#7477=DIRECTION ( 'NONE',  ( 1.156482317317869999E-16, 0.000000000000000000, 1.000000000000000000 ) ) ;
#7484=CARTESIAN_POINT ( 'NONE',  ( -57.08002265617300708, 84.22855780814606419, -15.00000000000001421 ) ) ;
#7487=ORIENTED_EDGE ( 'NONE', *, *, #1148, .F. ) ;
#7492=VECTOR ( 'NONE', #12970, 1000.000000000000000 ) ;
#7497=AXIS2_PLACEMENT_3D ( 'NONE', #14468, #16037, #14553 ) ;
#7504=CIRCLE ( 'NONE', #6008, 4.599999999999999645 ) ;
#7505=VERTEX_POINT ( 'NONE', #9308 ) ;
#7509=DIRECTION ( 'NONE',  ( 1.156482317317869999E-16, 0.000000000000000000, 1.000000000000000000 ) ) ;
#7524=ORIENTED_EDGE ( 'NONE', *, *, #17503, .T. ) ;
#7529=ORIENTED_EDGE ( 'NONE', *, *, #1497, .T. ) ;
#7530=CIRCLE ( 'NONE', #3637, 4.599999999999999645 ) ;
#7535=EDGE_CURVE ( 'NONE', #3299, #11538, #3328, .T. ) ;
#7537=AXIS2_PLACEMENT_3D ( 'NONE', #13749, #8134, #937 ) ;
#7538=FACE_OUTER_BOUND ( 'NONE', #13663, .T. ) ;
#7541=ORIENTED_EDGE ( 'NONE', *, *, #15095, .F. ) ;
#7555=LINE ( 'NONE', #1754, #8987 ) ;
#7561=AXIS2_PLACEMENT_3D ( 'NONE', #16612, #3805, #14919 ) ;
#7569=CIRCLE ( 'NONE', #1889, 4.599999999999992539 ) ;
#7575=DIRECTION ( 'NONE',  ( 1.000000000000000000, 0.000000000000000000, 5.077734830647309573E-16 ) ) ;
#7576=CARTESIAN_POINT ( 'NONE',  ( -49.40461175531926585, 94.09456345901895702, -15.00000000000001421 ) ) ;
#7578=CARTESIAN_POINT ( 'NONE',  ( -46.10942163047475617, 78.23723799236688592, -167.1454815528550739 ) ) ;
#7580=PRODUCT_DEFINITION_FORMATION_WITH_SPECIFIED_SOURCE ( 'ANY', '', #2532, .NOT_KNOWN. ) ;
#7600=AXIS2_PLACEMENT_3D ( 'NONE', #11892, #216, #5903 ) ;
#7601=ORIENTED_EDGE ( 'NONE', *, *, #13483, .F. ) ;
#7606=CARTESIAN_POINT ( 'NONE',  ( -57.08002265617300708, 84.22855780814606419, -167.1454815528550739 ) ) ;
#7617=EDGE_LOOP ( 'NONE', ( #6708, #947, #3797, #1472, #9023, #13946, #12032, #4433, #4128, #7280, #6118, #5618, #8335, #1100, #4592, #351, #8145, #1185, #13385, #14939, #4267, #16284, #4817, #3351, #11170, #12652, #15630, #13453, #5373, #8774, #11627, #14891, #12193, #12159, #8199, #12813, #14686, #13667, #6056, #2517, #643, #1374, #605, #4141, #9049, #18118, #8725, #17559, #578, #17382, #4842, #14609, #6680, #785, #7529, #12789, #14990, #1767, #17414, #8190, #6186, #8315, #13557, #3848, #3238, #12476, #15530, #18397, #15280, #14060, #9979, #2105, #1147, #2039, #15499, #13621, #149, #7784, #10946, #18095, #2349, #9392, #17402, #17210, #1808, #14545, #7817, #9089, #10623, #1109, #5188, #11915, #16590, #9994, #1592 ) ) ;
#7619=AXIS2_PLACEMENT_3D ( 'NONE', #11000, #14001, #16685 ) ;
#7621=CIRCLE ( 'NONE', #10916, 4.599999999999992539 ) ;
#7626=DIRECTION ( 'NONE',  ( -5.204170427930409450E-16, 0.000000000000000000, 1.000000000000000000 ) ) ;
#7627=DIRECTION ( 'NONE',  ( 1.000000000000000000, 0.000000000000000000, 0.000000000000000000 ) ) ;
#7634=ORIENTED_EDGE ( 'NONE', *, *, #17708, .F. ) ;
#7635=CIRCLE ( 'NONE', #7931, 4.599999999999999645 ) ;
#7639=EDGE_LOOP ( 'NONE', ( #9375, #10956, #2585, #6009 ) ) ;
#7640=VERTEX_POINT ( 'NONE', #1912 ) ;
#7665=EDGE_CURVE ( 'NONE', #12461, #10347, #13610, .T. ) ;
#7669=CARTESIAN_POINT ( 'NONE',  ( -64.89435165812551531, 90.86016871721213306, -15.00000000000001243 ) ) ;
#7682=ADVANCED_FACE ( 'NONE', ( #6476 ), #12198, .T. ) ;
#7685=DIRECTION ( 'NONE',  ( -1.000000000000000000, -1.624875145807134646E-14, 1.692578276882432005E-16 ) ) ;
#7699=DIRECTION ( 'NONE',  ( 0.000000000000000000, 0.000000000000000000, 1.000000000000000000 ) ) ;
#7715=CIRCLE ( 'NONE', #7145, 4.600000000000006750 ) ;
#7723=VERTEX_POINT ( 'NONE', #18282 ) ;
#7725=DIRECTION ( 'NONE',  ( 1.000000000000000000, 0.000000000000000000, 0.000000000000000000 ) ) ;
#7726=DIRECTION ( 'NONE',  ( 0.000000000000000000, 0.000000000000000000, 1.000000000000000000 ) ) ;
#7728=CYLINDRICAL_SURFACE ( 'NONE', #3115, 4.599999999999992539 ) ;
#7732=CYLINDRICAL_SURFACE ( 'NONE', #11542, 12.50000000000000355 ) ;
#7737=CARTESIAN_POINT ( 'NONE',  ( -57.08002265617300708, 84.22855780814606419, 15.00000000000006928 ) ) ;
#7740=CYLINDRICAL_SURFACE ( 'NONE', #4493, 7.500000000000000000 ) ;
#7741=DIRECTION ( 'NONE',  ( 0.000000000000000000, 0.000000000000000000, 1.000000000000000000 ) ) ;
#7743=AXIS2_PLACEMENT_3D ( 'NONE', #3306, #7626, #62 ) ;
#7750=EDGE_CURVE ( 'NONE', #14710, #2889, #11438, .T. ) ;
#7767=CARTESIAN_POINT ( 'NONE',  ( -66.35137518009933899, 89.78028827820979529, 15.00000000000006928 ) ) ;
#7780=EDGE_CURVE ( 'NONE', #12181, #11983, #6328, .T. ) ;
#7784=ORIENTED_EDGE ( 'NONE', *, *, #577, .T. ) ;
#7788=CARTESIAN_POINT ( 'NONE',  ( -67.79562744116532258, 82.83016482797231106, 15.00000000000006928 ) ) ;
#7793=ADVANCED_FACE ( 'NONE', ( #18473 ), #2468, .T. ) ;
#7817=ORIENTED_EDGE ( 'NONE', *, *, #469, .T. ) ;
#7828=CIRCLE ( 'NONE', #14687, 4.599999999999999645 ) ;
#7843=CIRCLE ( 'NONE', #6959, 12.50000000000000355 ) ;
#7851=DIRECTION ( 'NONE',  ( 0.000000000000000000, 0.000000000000000000, 1.000000000000000000 ) ) ;
#7856=VECTOR ( 'NONE', #5443, 1000.000000000000000 ) ;
#7866=AXIS2_PLACEMENT_3D ( 'NONE', #11568, #10342, #3222 ) ;
#7867=AXIS2_PLACEMENT_3D ( 'NONE', #2383, #15198, #1102 ) ;
#7870=FACE_OUTER_BOUND ( 'NONE', #9159, .T. ) ;
#7889=ORIENTED_EDGE ( 'NONE', *, *, #548, .T. ) ;
#7907=DIRECTION ( 'NONE',  ( -5.204170427930409450E-16, 0.000000000000000000, 1.000000000000000000 ) ) ;
#7910=AXIS2_PLACEMENT_3D ( 'NONE', #3653, #4766, #567 ) ;
#7912=AXIS2_PLACEMENT_3D ( 'NONE', #431, #12901, #12996 ) ;
#7923=CARTESIAN_POINT ( 'NONE',  ( -64.75543355702687620, 94.09456345901884333, 15.00000000000006928 ) ) ;
#7931=AXIS2_PLACEMENT_3D ( 'NONE', #6321, #17748, #7462 ) ;
#7932=FACE_OUTER_BOUND ( 'NONE', #8870, .T. ) ;
#7939=EDGE_LOOP ( 'NONE', ( #5993, #7889, #10359, #6886 ) ) ;
#7950=DIRECTION ( 'NONE',  ( -5.204170427930409450E-16, 0.000000000000000000, 1.000000000000000000 ) ) ;
#7951=CARTESIAN_POINT ( 'NONE',  ( -66.35137518009933899, 89.78028827820979529, -167.1454815528550739 ) ) ;
#7956=ORIENTED_EDGE ( 'NONE', *, *, #5023, .F. ) ;
#7968=CARTESIAN_POINT ( 'NONE',  ( -53.44605150580733266, 72.26844686893191749, -167.1454815528550739 ) ) ;
#7969=DIRECTION ( 'NONE',  ( 1.156482317317869999E-16, 0.000000000000000000, 1.000000000000000000 ) ) ;
#7980=ORIENTED_EDGE ( 'NONE', *, *, #18089, .F. ) ;
#7984=ORIENTED_EDGE ( 'NONE', *, *, #469, .F. ) ;
#7996=ORIENTED_EDGE ( 'NONE', *, *, #489, .T. ) ;
#7997=CIRCLE ( 'NONE', #841, 4.599999999999999645 ) ;
#8003=DIRECTION ( 'NONE',  ( 0.000000000000000000, 0.000000000000000000, 1.000000000000000000 ) ) ;
#8019=DIRECTION ( 'NONE',  ( 1.000000000000000000, 0.000000000000000000, 0.000000000000000000 ) ) ;
#8023=CIRCLE ( 'NONE', #8635, 4.599999999999999645 ) ;
#8029=FACE_OUTER_BOUND ( 'NONE', #97, .T. ) ;
#8030=FACE_OUTER_BOUND ( 'NONE', #12464, .T. ) ;
#8041=CARTESIAN_POINT ( 'NONE',  ( -57.08002265617300708, 84.22855780814606419, -15.00000000000001421 ) ) ;
#8043=ORIENTED_EDGE ( 'NONE', *, *, #10762, .F. ) ;
#8045=FACE_OUTER_BOUND ( 'NONE', #8690, .T. ) ;
#8047=AXIS2_PLACEMENT_3D ( 'NONE', #4263, #147, #5654 ) ;
#8048=DIRECTION ( 'NONE',  ( -5.204170427930409450E-16, 0.000000000000000000, 1.000000000000000000 ) ) ;
#8051=AXIS2_PLACEMENT_3D ( 'NONE', #15649, #2922, #18462 ) ;
#8053=ORIENTED_EDGE ( 'NONE', *, *, #8346, .T. ) ;
#8068=DIRECTION ( 'NONE',  ( -5.204170427930409450E-16, 0.000000000000000000, 1.000000000000000000 ) ) ;
#8077=DIRECTION ( 'NONE',  ( 1.000000000000000000, 0.000000000000000000, 0.000000000000000000 ) ) ;
#8079=DIRECTION ( 'NONE',  ( 0.000000000000000000, 0.000000000000000000, 1.000000000000000000 ) ) ;
#8090=CIRCLE ( 'NONE', #10482, 10.24900000000000055 ) ;
#8095=LINE ( 'NONE', #5297, #13766 ) ;
#8099=VERTEX_POINT ( 'NONE', #14793 ) ;
#8102=CARTESIAN_POINT ( 'NONE',  ( -60.62932119839002354, 94.43552448259767118, -167.1454815528550739 ) ) ;
#8103=CARTESIAN_POINT ( 'NONE',  ( -48.21445538031289857, 89.37090336996882911, -15.00000000000001421 ) ) ;
#8109=AXIS2_PLACEMENT_3D ( 'NONE', #13017, #191, #10370 ) ;
#8111=CARTESIAN_POINT ( 'NONE',  ( -55.64822083176820655, 96.64628479562776420, 15.00000000000006928 ) ) ;
#8113=EDGE_LOOP ( 'NONE', ( #683, #16919, #435, #9515 ) ) ;
#8115=EDGE_CURVE ( 'NONE', #16289, #16963, #2175, .T. ) ;
#8121=AXIS2_PLACEMENT_3D ( 'NONE', #4632, #17347, #6022 ) ;
#8127=CARTESIAN_POINT ( 'NONE',  ( -47.76628296033400289, 88.50596986196467242, -167.1454815528550739 ) ) ;
#8134=DIRECTION ( 'NONE',  ( 1.156482317317869999E-16, 0.000000000000000000, 1.000000000000000000 ) ) ;
#8140=ORIENTED_EDGE ( 'NONE', *, *, #6429, .F. ) ;
#8141=CIRCLE ( 'NONE', #8754, 7.500000000000000000 ) ;
#8144=CARTESIAN_POINT ( 'NONE',  ( -57.08002265617300708, 84.22855780814606419, 15.00000000000006928 ) ) ;
#8145=ORIENTED_EDGE ( 'NONE', *, *, #466, .T. ) ;
#8149=VERTEX_POINT ( 'NONE', #18164 ) ;
#8155=AXIS2_PLACEMENT_3D ( 'NONE', #1770, #7477, #9171 ) ;
#8168=AXIS2_PLACEMENT_3D ( 'NONE', #3992, #16990, #7089 ) ;
#8176=DIRECTION ( 'NONE',  ( 1.000000000000000000, 0.000000000000000000, 3.771137991253928573E-16 ) ) ;
#8190=ORIENTED_EDGE ( 'NONE', *, *, #17104, .T. ) ;
#8199=ORIENTED_EDGE ( 'NONE', *, *, #17595, .T. ) ;
#8209=DIRECTION ( 'NONE',  ( 1.156482317317869999E-16, 0.000000000000000000, 1.000000000000000000 ) ) ;
#8214=CIRCLE ( 'NONE', #7912, 4.600000000000006750 ) ;
#8215=CIRCLE ( 'NONE', #1073, 12.49999999999999645 ) ;
#8217=FACE_OUTER_BOUND ( 'NONE', #9982, .T. ) ;
#8225=VECTOR ( 'NONE', #12418, 1000.000000000000000 ) ;
#8227=AXIS2_PLACEMENT_3D ( 'NONE', #11947, #10451, #3337 ) ;
#8236=CARTESIAN_POINT ( 'NONE',  ( -56.80760832784252301, 71.73152654333280509, -15.00000000000001421 ) ) ;
#8274=CARTESIAN_POINT ( 'NONE',  ( -53.39175999306721110, 74.07097899412303832, -15.00000000000001421 ) ) ;
#8279=EDGE_LOOP ( 'NONE', ( #15535, #12035, #2203, #14104 ) ) ;
#8282=ORIENTED_EDGE ( 'NONE', *, *, #4989, .T. ) ;
#8283=DIRECTION ( 'NONE',  ( -5.204170427930409450E-16, 0.000000000000000000, 1.000000000000000000 ) ) ;
#8289=ORIENTED_EDGE ( 'NONE', *, *, #7062, .F. ) ;
#8297=DIRECTION ( 'NONE',  ( -1.000000000000000000, 3.330669073875471988E-15, 1.387778780781446662E-16 ) ) ;
#8299=CARTESIAN_POINT ( 'NONE',  ( -65.72457281170906640, 78.72276507608454210, -15.00000000000001421 ) ) ;
#8306=CYLINDRICAL_SURFACE ( 'NONE', #1051, 12.49999999999999112 ) ;
#8315=ORIENTED_EDGE ( 'NONE', *, *, #14291, .T. ) ;
#8332=CIRCLE ( 'NONE', #13399, 10.24900000000001477 ) ;
#8334=EDGE_CURVE ( 'NONE', #15321, #4520, #15317, .T. ) ;
#8335=ORIENTED_EDGE ( 'NONE', *, *, #8719, .T. ) ;
#8346=EDGE_CURVE ( 'NONE', #11711, #197, #6048, .T. ) ;
#8354=ORIENTED_EDGE ( 'NONE', *, *, #8360, .F. ) ;
#8360=EDGE_CURVE ( 'NONE', #6937, #11248, #3330, .T. ) ;
#8365=DIRECTION ( 'NONE',  ( -5.204170427930409450E-16, 0.000000000000000000, 1.000000000000000000 ) ) ;
#8373=FACE_OUTER_BOUND ( 'NONE', #15153, .T. ) ;
#8374=EDGE_CURVE ( 'NONE', #15261, #14168, #9350, .T. ) ;
#8377=VERTEX_POINT ( 'NONE', #16240 ) ;
#8394=DIRECTION ( 'NONE',  ( 0.000000000000000000, 0.000000000000000000, 1.000000000000000000 ) ) ;
#8395=CARTESIAN_POINT ( 'NONE',  ( -54.78701292294434211, 94.21775734381050427, 15.00000000000006928 ) ) ;
#8397=LINE ( 'NONE', #15303, #104 ) ;
#8402=DIRECTION ( 'NONE',  ( -1.000000000000000000, 3.016910393003138520E-15, 0.000000000000000000 ) ) ;
#8405=CIRCLE ( 'NONE', #17046, 12.49999999999999112 ) ;
#8411=DIRECTION ( 'NONE',  ( 1.000000000000000000, 0.000000000000000000, 5.551115123125784674E-16 ) ) ;
#8421=DIRECTION ( 'NONE',  ( 1.000000000000000000, 0.000000000000000000, 5.551115123125777772E-16 ) ) ;
#8428=ORIENTED_EDGE ( 'NONE', *, *, #8594, .T. ) ;
#8430=AXIS2_PLACEMENT_3D ( 'NONE', #11267, #10038, #5894 ) ;
#8433=ORIENTED_EDGE ( 'NONE', *, *, #815, .T. ) ;
#8434=ORIENTED_EDGE ( 'NONE', *, *, #10037, .F. ) ;
#8437=VERTEX_POINT ( 'NONE', #14569 ) ;
#8440=CARTESIAN_POINT ( 'NONE',  ( -64.22944241949029731, 91.57211267264378307, 15.00000000000006928 ) ) ;
#8462=DIRECTION ( 'NONE',  ( 1.000000000000000000, 0.000000000000000000, 0.000000000000000000 ) ) ;
#8470=CYLINDRICAL_SURFACE ( 'NONE', #6593, 10.24900000000000055 ) ;
#8471=CARTESIAN_POINT ( 'NONE',  ( -49.26569365422058411, 90.86016871721223254, -167.1454815528550739 ) ) ;
#8475=DIRECTION ( 'NONE',  ( 1.156482317317869999E-16, 0.000000000000000000, 1.000000000000000000 ) ) ;
#8477=EDGE_CURVE ( 'NONE', #14981, #11552, #12341, .T. ) ;
#8481=AXIS2_PLACEMENT_3D ( 'NONE', #16716, #12537, #18235 ) ;
#8482=ORIENTED_EDGE ( 'NONE', *, *, #717, .T. ) ;
#8486=EDGE_CURVE ( 'NONE', #2327, #10261, #3892, .T. ) ;
#8489=FACE_OUTER_BOUND ( 'NONE', #5291, .T. ) ;
#8507=EDGE_CURVE ( 'NONE', #9948, #1399, #18021, .T. ) ;
#8510=EDGE_CURVE ( 'NONE', #1656, #1289, #2117, .T. ) ;
#8513=CARTESIAN_POINT ( 'NONE',  ( -57.08002265617300708, 84.22855780814606419, -167.1454815528550739 ) ) ;
#8514=ORIENTED_EDGE ( 'NONE', *, *, #10844, .F. ) ;
#8519=AXIS2_PLACEMENT_3D ( 'NONE', #1439, #13890, #1085 ) ;
#8523=FACE_BOUND ( 'NONE', #321, .T. ) ;
#8527=CIRCLE ( 'NONE', #12406, 4.599999999999992539 ) ;
#8541=AXIS2_PLACEMENT_3D ( 'NONE', #16832, #6633, #9736 ) ;
#8548=ORIENTED_EDGE ( 'NONE', *, *, #14867, .F. ) ;
#8553=AXIS2_PLACEMENT_3D ( 'NONE', #18130, #16703, #11218 ) ;
#8554=AXIS2_PLACEMENT_3D ( 'NONE', #3897, #12524, #9605 ) ;
#8556=VERTEX_POINT ( 'NONE', #12327 ) ;
#8562=ORIENTED_EDGE ( 'NONE', *, *, #12728, .T. ) ;
#8565=ORIENTED_EDGE ( 'NONE', *, *, #6255, .F. ) ;
#8566=LINE ( 'NONE', #5561, #7492 ) ;
#8576=FACE_OUTER_BOUND ( 'NONE', #7639, .T. ) ;
#8579=DIRECTION ( 'NONE',  ( -1.000000000000000000, 0.000000000000000000, 0.000000000000000000 ) ) ;
#8580=ORIENTED_EDGE ( 'NONE', *, *, #952, .F. ) ;
#8589=ORIENTED_EDGE ( 'NONE', *, *, #2652, .T. ) ;
#8591=EDGE_CURVE ( 'NONE', #12513, #1656, #3981, .T. ) ;
#8592=CARTESIAN_POINT ( 'NONE',  ( -58.95655619609375009, 74.15281352429524020, 15.00000000000006928 ) ) ;
#8594=EDGE_CURVE ( 'NONE', #1045, #7123, #15336, .T. ) ;
#8602=ORIENTED_EDGE ( 'NONE', *, *, #2385, .T. ) ;
#8604=CARTESIAN_POINT ( 'NONE',  ( -68.76426085488260753, 88.67024416760638417, 15.00000000000006928 ) ) ;
#8614=EDGE_CURVE ( 'NONE', #18335, #14903, #16209, .T. ) ;
#8615=EDGE_CURVE ( 'NONE', #6278, #2307, #8397, .T. ) ;
#8617=ORIENTED_EDGE ( 'NONE', *, *, #1525, .F. ) ;
#8618=DIRECTION ( 'NONE',  ( 1.156482317317869999E-16, 0.000000000000000000, 1.000000000000000000 ) ) ;
#8627=DIRECTION ( 'NONE',  ( 0.000000000000000000, 0.000000000000000000, 1.000000000000000000 ) ) ;
#8634=DIRECTION ( 'NONE',  ( -1.000000000000000000, 3.016910393003138520E-15, 0.000000000000000000 ) ) ;
#8635=AXIS2_PLACEMENT_3D ( 'NONE', #3835, #5327, #16843 ) ;
#8640=CARTESIAN_POINT ( 'NONE',  ( -59.20641439073742873, 73.63336328296978195, 15.00000000000006928 ) ) ;
#8642=DIRECTION ( 'NONE',  ( -1.000000000000000000, 2.220446049250309925E-14, 1.387778780781443703E-16 ) ) ;
#8649=DIRECTION ( 'NONE',  ( 1.156482317317869999E-16, 0.000000000000000000, 1.000000000000000000 ) ) ;
#8654=AXIS2_PLACEMENT_3D ( 'NONE', #12190, #16383, #10607 ) ;
#8658=EDGE_LOOP ( 'NONE', ( #6231, #17721, #14811, #16303 ) ) ;
#8662=CARTESIAN_POINT ( 'NONE',  ( -67.44681693414594292, 91.21279551874751235, -15.00000000000001243 ) ) ;
#8669=AXIS2_PLACEMENT_3D ( 'NONE', #7431, #11991, #10597 ) ;
#8674=EDGE_CURVE ( 'NONE', #6741, #2018, #17183, .T. ) ;
#8690=EDGE_LOOP ( 'NONE', ( #15526, #7318, #11840, #6087 ) ) ;
#8697=AXIS2_PLACEMENT_3D ( 'NONE', #2329, #2536, #16840 ) ;
#8700=ADVANCED_FACE ( 'NONE', ( #1819 ), #4707, .T. ) ;
#8706=CARTESIAN_POINT ( 'NONE',  ( -68.94671286412481948, 88.15687341518439268, 15.00000000000006928 ) ) ;
#8711=ORIENTED_EDGE ( 'NONE', *, *, #12727, .F. ) ;
#8713=AXIS2_PLACEMENT_3D ( 'NONE', #18480, #11374, #11470 ) ;
#8718=CARTESIAN_POINT ( 'NONE',  ( -59.05157857372951469, 96.57209730311865314, -167.1454815528550739 ) ) ;
#8719=EDGE_CURVE ( 'NONE', #8972, #9420, #10200, .T. ) ;
#8723=ADVANCED_FACE ( 'NONE', ( #3307 ), #9030, .T. ) ;
#8724=DIRECTION ( 'NONE',  ( 1.000000000000000000, 0.000000000000000000, 0.000000000000000000 ) ) ;
#8725=ORIENTED_EDGE ( 'NONE', *, *, #4933, .T. ) ;
#8728=CARTESIAN_POINT ( 'NONE',  ( -67.50540723371459251, 87.07303407725210320, -15.00000000000001421 ) ) ;
#8742=CIRCLE ( 'NONE', #16488, 4.599999999999999645 ) ;
#8750=CARTESIAN_POINT ( 'NONE',  ( -50.90853507983961634, 93.09943318379598054, -167.1454815528550739 ) ) ;
#8751=ORIENTED_EDGE ( 'NONE', *, *, #17610, .F. ) ;
#8753=VERTEX_POINT ( 'NONE', #15953 ) ;
#8754=AXIS2_PLACEMENT_3D ( 'NONE', #15155, #4965, #11985 ) ;
#8771=AXIS2_PLACEMENT_3D ( 'NONE', #11317, #1481, #13937 ) ;
#8774=ORIENTED_EDGE ( 'NONE', *, *, #7750, .T. ) ;
#8776=CARTESIAN_POINT ( 'NONE',  ( -66.96222586426215173, 88.60139997190893268, 15.00000000000006928 ) ) ;
#8780=AXIS2_PLACEMENT_3D ( 'NONE', #999, #9887, #8579 ) ;
#8782=DIRECTION ( 'NONE',  ( 0.000000000000000000, 0.000000000000000000, 1.000000000000000000 ) ) ;
#8783=DIRECTION ( 'NONE',  ( 0.000000000000000000, 0.000000000000000000, 1.000000000000000000 ) ) ;
#8784=DIRECTION ( 'NONE',  ( 1.156482317317869999E-16, 0.000000000000000000, 1.000000000000000000 ) ) ;
#8795=CIRCLE ( 'NONE', #3117, 12.50000000000000355 ) ;
#8807=CIRCLE ( 'NONE', #4333, 10.24899999999998812 ) ;
#8808=CARTESIAN_POINT ( 'NONE',  ( -65.17806329749801364, 93.75072866207683830, 15.00000000000006928 ) ) ;
#8812=ADVANCED_FACE ( 'NONE', ( #8859 ), #3048, .T. ) ;
#8816=CIRCLE ( 'NONE', #5529, 10.24900000000000766 ) ;
#8837=AXIS2_PLACEMENT_3D ( 'NONE', #2123, #13181, #13546 ) ;
#8839=AXIS2_PLACEMENT_3D ( 'NONE', #2395, #5303, #2304 ) ;
#8842=EDGE_LOOP ( 'NONE', ( #3624, #8562, #13103, #2707 ) ) ;
#8847=ORIENTED_EDGE ( 'NONE', *, *, #2041, .F. ) ;
#8851=ORIENTED_EDGE ( 'NONE', *, *, #4689, .T. ) ;
#8852=CIRCLE ( 'NONE', #17790, 12.49999999999999112 ) ;
#8859=FACE_OUTER_BOUND ( 'NONE', #16519, .T. ) ;
#8862=CARTESIAN_POINT ( 'NONE',  ( -61.60537251683745552, 75.03273214436880778, -167.1454815528550739 ) ) ;
#8866=DIRECTION ( 'NONE',  ( 1.000000000000000000, 0.000000000000000000, 3.771137991253934490E-16 ) ) ;
#8867=CARTESIAN_POINT ( 'NONE',  ( -67.00421887699711476, 86.78830982163884755, -15.00000000000001421 ) ) ;
#8870=EDGE_LOOP ( 'NONE', ( #9950, #11463, #5055, #6786 ) ) ;
#8878=ORIENTED_EDGE ( 'NONE', *, *, #15337, .T. ) ;
#8882=DIRECTION ( 'NONE',  ( 0.000000000000000000, 0.000000000000000000, 1.000000000000000000 ) ) ;
#8901=CARTESIAN_POINT ( 'NONE',  ( -57.08002265617300708, 84.22855780814606419, -15.00000000000001421 ) ) ;
#8902=CARTESIAN_POINT ( 'NONE',  ( -58.95655619609375009, 74.15281352429524020, -167.1454815528550739 ) ) ;
#8910=DIRECTION ( 'NONE',  ( -1.000000000000000000, 1.354062621505947576E-15, 1.692578276882434470E-16 ) ) ;
#8914=EDGE_CURVE ( 'NONE', #2040, #2137, #4517, .T. ) ;
#8915=ORIENTED_EDGE ( 'NONE', *, *, #1025, .T. ) ;
#8927=ADVANCED_FACE ( 'NONE', ( #6292 ), #9403, .T. ) ;
#8933=CARTESIAN_POINT ( 'NONE',  ( -44.78895386838529902, 81.95267818613812949, 15.00000000000006928 ) ) ;
#8935=VERTEX_POINT ( 'NONE', #5076 ) ;
#8938=DIRECTION ( 'NONE',  ( -5.204170427930409450E-16, 0.000000000000000000, 1.000000000000000000 ) ) ;
#8949=DIRECTION ( 'NONE',  ( 0.000000000000000000, 0.000000000000000000, 1.000000000000000000 ) ) ;
#8954=ORIENTED_EDGE ( 'NONE', *, *, #6432, .F. ) ;
#8956=CIRCLE ( 'NONE', #8047, 4.599999999999992539 ) ;
#8957=FACE_OUTER_BOUND ( 'NONE', #12271, .T. ) ;
#8960=DIRECTION ( 'NONE',  ( 1.000000000000000000, 0.000000000000000000, 0.000000000000000000 ) ) ;
#8961=DIRECTION ( 'NONE',  ( 1.000000000000000000, 0.000000000000000000, 0.000000000000000000 ) ) ;
#8972=VERTEX_POINT ( 'NONE', #16967 ) ;
#8980=ORIENTED_EDGE ( 'NONE', *, *, #5612, .T. ) ;
#8981=CARTESIAN_POINT ( 'NONE',  ( -63.80603561266293156, 73.69239390902558284, -15.00000000000001421 ) ) ;
#8987=VECTOR ( 'NONE', #17206, 1000.000000000000000 ) ;
#8998=AXIS2_PLACEMENT_3D ( 'NONE', #10228, #12693, #14272 ) ;
#9000=DIRECTION ( 'NONE',  ( -5.204170427930409450E-16, 0.000000000000000000, 1.000000000000000000 ) ) ;
#9001=ORIENTED_EDGE ( 'NONE', *, *, #8374, .F. ) ;
#9004=ORIENTED_EDGE ( 'NONE', *, *, #12014, .F. ) ;
#9006=LINE ( 'NONE', #669, #14185 ) ;
#9011=CARTESIAN_POINT ( 'NONE',  ( -49.65031598894605480, 92.07579602767992810, -167.1454815528550739 ) ) ;
#9023=ORIENTED_EDGE ( 'NONE', *, *, #3446, .T. ) ;
#9030=CYLINDRICAL_SURFACE ( 'NONE', #14099, 4.599999999999992539 ) ;
#9049=ORIENTED_EDGE ( 'NONE', *, *, #17169, .T. ) ;
#9050=FACE_OUTER_BOUND ( 'NONE', #13955, .T. ) ;
#9053=CIRCLE ( 'NONE', #2483, 4.599999999999992539 ) ;
#9054=DIRECTION ( 'NONE',  ( 0.000000000000000000, 0.000000000000000000, 1.000000000000000000 ) ) ;
#9056=DIRECTION ( 'NONE',  ( 0.000000000000000000, 0.000000000000000000, 1.000000000000000000 ) ) ;
#9057=ORIENTED_EDGE ( 'NONE', *, *, #17130, .T. ) ;
#9066=AXIS2_PLACEMENT_3D ( 'NONE', #7170, #11211, #15497 ) ;
#9067=DIRECTION ( 'NONE',  ( 0.000000000000000000, 0.000000000000000000, 1.000000000000000000 ) ) ;
#9072=VERTEX_POINT ( 'NONE', #15073 ) ;
#9077=CARTESIAN_POINT ( 'NONE',  ( -56.41614838398844256, 95.01461175692088545, 15.00000000000006928 ) ) ;
#9082=FACE_OUTER_BOUND ( 'NONE', #5429, .T. ) ;
#9084=CARTESIAN_POINT ( 'NONE',  ( -49.75809927370887920, 76.28065702765852052, -167.1454815528550739 ) ) ;
#9085=ORIENTED_EDGE ( 'NONE', *, *, #10743, .F. ) ;
#9089=ORIENTED_EDGE ( 'NONE', *, *, #4376, .T. ) ;
#9091=DIRECTION ( 'NONE',  ( 1.156482317317869999E-16, 0.000000000000000000, 1.000000000000000000 ) ) ;
#9095=AXIS2_PLACEMENT_3D ( 'NONE', #10076, #14372, #16903 ) ;
#9105=CIRCLE ( 'NONE', #154, 4.599999999999992539 ) ;
#9117=ORIENTED_EDGE ( 'NONE', *, *, #3534, .T. ) ;
#9119=CIRCLE ( 'NONE', #5542, 10.24900000000000055 ) ;
#9120=VECTOR ( 'NONE', #9054, 1000.000000000000000 ) ;
#9122=ORIENTED_EDGE ( 'NONE', *, *, #577, .F. ) ;
#9140=CARTESIAN_POINT ( 'NONE',  ( -63.16290507965269541, 75.97988867778799715, 15.00000000000006928 ) ) ;
#9142=ORIENTED_EDGE ( 'NONE', *, *, #15442, .T. ) ;
#9144=CARTESIAN_POINT ( 'NONE',  ( -64.40194603863702127, 76.28065702765842104, -167.1454815528550739 ) ) ;
#9145=DIRECTION ( 'NONE',  ( -1.000000000000000000, 0.000000000000000000, 0.000000000000000000 ) ) ;
#9150=DIRECTION ( 'NONE',  ( 0.000000000000000000, 0.000000000000000000, 1.000000000000000000 ) ) ;
#9159=EDGE_LOOP ( 'NONE', ( #12908, #17004, #1488, #16898 ) ) ;
#9161=EDGE_CURVE ( 'NONE', #4200, #274, #3042, .T. ) ;
#9162=DIRECTION ( 'NONE',  ( 0.000000000000000000, 0.000000000000000000, 1.000000000000000000 ) ) ;
#9171=DIRECTION ( 'NONE',  ( -1.000000000000000000, 0.000000000000000000, 0.000000000000000000 ) ) ;
#9178=ORIENTED_EDGE ( 'NONE', *, *, #6283, .F. ) ;
#9182=ORIENTED_EDGE ( 'NONE', *, *, #11444, .F. ) ;
#9184=DIRECTION ( 'NONE',  ( 1.156482317317869999E-16, 0.000000000000000000, 1.000000000000000000 ) ) ;
#9189=CARTESIAN_POINT ( 'NONE',  ( -66.27474722583565381, 78.55081803573735044, -15.00000000000001421 ) ) ;
#9195=ORIENTED_EDGE ( 'NONE', *, *, #11899, .F. ) ;
#9204=VERTEX_POINT ( 'NONE', #15260 ) ;
#9208=DIRECTION ( 'NONE',  ( 0.000000000000000000, 0.000000000000000000, 1.000000000000000000 ) ) ;
#9220=CIRCLE ( 'NONE', #11335, 10.24900000000000055 ) ;
#9222=VERTEX_POINT ( 'NONE', #2449 ) ;
#9224=DIRECTION ( 'NONE',  ( 1.156482317317869999E-16, 0.000000000000000000, 1.000000000000000000 ) ) ;
#9225=DIRECTION ( 'NONE',  ( 1.000000000000000000, 0.000000000000000000, 3.771137991253923150E-16 ) ) ;
#9234=CARTESIAN_POINT ( 'NONE',  ( -57.08002265617300708, 84.22855780814606419, -167.1454815528550739 ) ) ;
#9246=ORIENTED_EDGE ( 'NONE', *, *, #4678, .T. ) ;
#9250=VERTEX_POINT ( 'NONE', #6843 ) ;
#9259=AXIS2_PLACEMENT_3D ( 'NONE', #21, #10122, #15827 ) ;
#9266=CARTESIAN_POINT ( 'NONE',  ( -57.08002265617300708, 84.22855780814606419, -15.00000000000001421 ) ) ;
#9272=ORIENTED_EDGE ( 'NONE', *, *, #10900, .T. ) ;
#9278=DIRECTION ( 'NONE',  ( 0.000000000000000000, 0.000000000000000000, 1.000000000000000000 ) ) ;
#9282=CARTESIAN_POINT ( 'NONE',  ( -58.95655619609375009, 74.15281352429524020, -15.00000000000001421 ) ) ;
#9284=VERTEX_POINT ( 'NONE', #9940 ) ;
#9286=CYLINDRICAL_SURFACE ( 'NONE', #11712, 12.50000000000001066 ) ;
#9290=ADVANCED_FACE ( 'NONE', ( #10035 ), #5808, .T. ) ;
#9307=VERTEX_POINT ( 'NONE', #2836 ) ;
#9308=CARTESIAN_POINT ( 'NONE',  ( -47.76080550507955280, 75.89776002577458769, 15.00000000000006928 ) ) ;
#9319=CYLINDRICAL_SURFACE ( 'NONE', #3390, 12.49999999999999112 ) ;
#9322=CIRCLE ( 'NONE', #13216, 12.49999999999999112 ) ;
#9335=CARTESIAN_POINT ( 'NONE',  ( -57.35243698450333483, 71.73152654333280509, -167.1454815528550739 ) ) ;
#9340=DIRECTION ( 'NONE',  ( -1.000000000000000000, 0.000000000000000000, 1.387778780781446662E-16 ) ) ;
#9346=ORIENTED_EDGE ( 'NONE', *, *, #8477, .T. ) ;
#9350=CIRCLE ( 'NONE', #1308, 4.600000000000006750 ) ;
#9354=VERTEX_POINT ( 'NONE', #7133 ) ;
#9366=VERTEX_POINT ( 'NONE', #15741 ) ;
#9375=ORIENTED_EDGE ( 'NONE', *, *, #8615, .F. ) ;
#9377=DIRECTION ( 'NONE',  ( -5.204170427930409450E-16, 0.000000000000000000, 1.000000000000000000 ) ) ;
#9392=ORIENTED_EDGE ( 'NONE', *, *, #4698, .T. ) ;
#9393=AXIS2_PLACEMENT_3D ( 'NONE', #8274, #11363, #11276 ) ;
#9397=CARTESIAN_POINT ( 'NONE',  ( -69.56651066787533466, 84.80960611389535586, 15.00000000000006928 ) ) ;
#9400=VERTEX_POINT ( 'NONE', #4671 ) ;
#9403=CYLINDRICAL_SURFACE ( 'NONE', #13783, 10.24900000000000766 ) ;
#9406=ADVANCED_FACE ( 'NONE', ( #2243 ), #14777, .T. ) ;
#9411=CYLINDRICAL_SURFACE ( 'NONE', #9932, 4.599999999999992539 ) ;
#9418=AXIS2_PLACEMENT_3D ( 'NONE', #18236, #5598, #16923 ) ;
#9420=VERTEX_POINT ( 'NONE', #11878 ) ;
#9427=ORIENTED_EDGE ( 'NONE', *, *, #10135, .F. ) ;
#9428=DIRECTION ( 'NONE',  ( 0.000000000000000000, 0.000000000000000000, 1.000000000000000000 ) ) ;
#9429=DIRECTION ( 'NONE',  ( 1.000000000000000000, 0.000000000000000000, 3.771137991253934490E-16 ) ) ;
#9432=CARTESIAN_POINT ( 'NONE',  ( -57.08002265617300708, 84.22855780814606419, -167.1454815528550739 ) ) ;
#9440=VERTEX_POINT ( 'NONE', #16446 ) ;
#9444=DIRECTION ( 'NONE',  ( -5.204170427930409450E-16, 0.000000000000000000, 1.000000000000000000 ) ) ;
#9446=LINE ( 'NONE', #10746, #2493 ) ;
#9449=CARTESIAN_POINT ( 'NONE',  ( -47.76080550507955280, 75.89776002577458769, -167.1454815528550739 ) ) ;
#9457=VERTEX_POINT ( 'NONE', #4853 ) ;
#9460=DIRECTION ( 'NONE',  ( 1.156482317317869999E-16, 0.000000000000000000, 1.000000000000000000 ) ) ;
#9476=ADVANCED_FACE ( 'NONE', ( #13662 ), #12073, .T. ) ;
#9485=CARTESIAN_POINT ( 'NONE',  ( -57.08002265617300708, 84.22855780814606419, 15.00000000000006928 ) ) ;
#9488=ORIENTED_EDGE ( 'NONE', *, *, #7030, .T. ) ;
#9500=VERTEX_POINT ( 'NONE', #16167 ) ;
#9501=DIRECTION ( 'NONE',  ( 1.000000000000000000, 0.000000000000000000, 0.000000000000000000 ) ) ;
#9504=ADVANCED_FACE ( 'NONE', ( #3358 ), #14861, .T. ) ;
#9510=CYLINDRICAL_SURFACE ( 'NONE', #4783, 4.599999999999992539 ) ;
#9511=DIRECTION ( 'NONE',  ( -1.000000000000000000, -3.016910393003138520E-15, 0.000000000000000000 ) ) ;
#9515=ORIENTED_EDGE ( 'NONE', *, *, #7780, .F. ) ;
#9525=AXIS2_PLACEMENT_3D ( 'NONE', #12798, #5578, #8297 ) ;
#9531=CARTESIAN_POINT ( 'NONE',  ( -57.08002265617300708, 84.22855780814606419, -167.1454815528550739 ) ) ;
#9534=DIRECTION ( 'NONE',  ( -5.204170427930409450E-16, 0.000000000000000000, 1.000000000000000000 ) ) ;
#9537=EDGE_CURVE ( 'NONE', #2450, #7505, #7033, .T. ) ;
#9544=VERTEX_POINT ( 'NONE', #13945 ) ;
#9546=DIRECTION ( 'NONE',  ( 0.000000000000000000, 0.000000000000000000, 1.000000000000000000 ) ) ;
#9550=ADVANCED_FACE ( 'NONE', ( #10952 ), #17948, .T. ) ;
#9553=VECTOR ( 'NONE', #11161, 1000.000000000000000 ) ;
#9554=DIRECTION ( 'NONE',  ( 1.156482317317869999E-16, 0.000000000000000000, 1.000000000000000000 ) ) ;
#9556=CARTESIAN_POINT ( 'NONE',  ( -65.94558993203320085, 89.37090336996871542, -15.00000000000001421 ) ) ;
#9564=VERTEX_POINT ( 'NONE', #8236 ) ;
#9565=VECTOR ( 'NONE', #7230, 1000.000000000000000 ) ;
#9569=CARTESIAN_POINT ( 'NONE',  ( -64.58002265617299997, 84.22855780814606419, 15.00000000000006573 ) ) ;
#9572=ORIENTED_EDGE ( 'NONE', *, *, #17022, .F. ) ;
#9573=CIRCLE ( 'NONE', #1523, 4.599999999999992539 ) ;
#9583=CIRCLE ( 'NONE', #16135, 4.599999999999992539 ) ;
#9605=DIRECTION ( 'NONE',  ( 1.000000000000000000, 0.000000000000000000, 3.771137991253934490E-16 ) ) ;
#9617=ORIENTED_EDGE ( 'NONE', *, *, #6814, .F. ) ;
#9619=EDGE_CURVE ( 'NONE', #1231, #6109, #2457, .T. ) ;
#9632=CARTESIAN_POINT ( 'NONE',  ( -48.98198201484814263, 93.75072866207695199, -15.00000000000001421 ) ) ;
#9634=FACE_OUTER_BOUND ( 'NONE', #5968, .T. ) ;
#9637=EDGE_CURVE ( 'NONE', #15366, #15625, #3645, .T. ) ;
#9640=VERTEX_POINT ( 'NONE', #16635 ) ;
#9654=LINE ( 'NONE', #11536, #18234 ) ;
#9659=DIRECTION ( 'NONE',  ( 0.000000000000000000, 0.000000000000000000, 1.000000000000000000 ) ) ;
#9660=DIRECTION ( 'NONE',  ( 1.000000000000000000, 0.000000000000000000, 0.000000000000000000 ) ) ;
#9669=( GEOMETRIC_REPRESENTATION_CONTEXT ( 3 ) GLOBAL_UNCERTAINTY_ASSIGNED_CONTEXT ( ( #3473 ) ) GLOBAL_UNIT_ASSIGNED_CONTEXT ( ( #2021, #13439, #812 ) ) REPRESENTATION_CONTEXT ( 'NONE', 'WORKASPACE' ) );
#9673=CARTESIAN_POINT ( 'NONE',  ( -65.16279959635889441, 77.92691374209478283, -167.1454815528550739 ) ) ;
#9689=DIRECTION ( 'NONE',  ( 1.156482317317869999E-16, 0.000000000000000000, 1.000000000000000000 ) ) ;
#9696=ORIENTED_EDGE ( 'NONE', *, *, #17709, .T. ) ;
#9700=DIRECTION ( 'NONE',  ( 0.000000000000000000, 0.000000000000000000, 1.000000000000000000 ) ) ;
#9704=LINE ( 'NONE', #12428, #1198 ) ;
#9705=LINE ( 'NONE', #1192, #12221 ) ;
#9716=AXIS2_PLACEMENT_3D ( 'NONE', #5417, #15438, #2623 ) ;
#9736=DIRECTION ( 'NONE',  ( 1.000000000000000000, 0.000000000000000000, 0.000000000000000000 ) ) ;
#9745=CARTESIAN_POINT ( 'NONE',  ( -60.71187100093244737, 74.64462966772953223, 15.00000000000006928 ) ) ;
#9754=ADVANCED_FACE ( 'NONE', ( #92 ), #10277, .T. ) ;
#9755=EDGE_CURVE ( 'NONE', #18489, #16773, #11723, .T. ) ;
#9757=DIRECTION ( 'NONE',  ( -1.000000000000000000, 3.016910393003147592E-15, 0.000000000000000000 ) ) ;
#9763=DIRECTION ( 'NONE',  ( 1.000000000000000000, 0.000000000000000000, 3.771137991253923150E-16 ) ) ;
#9767=ORIENTED_EDGE ( 'NONE', *, *, #10844, .T. ) ;
#9771=ORIENTED_EDGE ( 'NONE', *, *, #14954, .T. ) ;
#9777=CARTESIAN_POINT ( 'NONE',  ( -54.95363092160842911, 73.63336328296981037, 15.00000000000006928 ) ) ;
#9798=ORIENTED_EDGE ( 'NONE', *, *, #6196, .T. ) ;
#9800=CARTESIAN_POINT ( 'NONE',  ( -65.50906076758114693, 77.46608744949911340, -15.00000000000001421 ) ) ;
#9810=DIRECTION ( 'NONE',  ( 0.000000000000000000, 0.000000000000000000, 1.000000000000000000 ) ) ;
#9819=ORIENTED_EDGE ( 'NONE', *, *, #1982, .F. ) ;
#9828=ADVANCED_FACE ( 'NONE', ( #15885 ), #14237, .T. ) ;
#9832=CIRCLE ( 'NONE', #15503, 4.600000000000006750 ) ;
#9834=EDGE_LOOP ( 'NONE', ( #2700, #13886, #9142, #5728 ) ) ;
#9840=ADVANCED_FACE ( 'NONE', ( #13272 ), #5284, .T. ) ;
#9845=DIRECTION ( 'NONE',  ( -1.000000000000000000, 4.062187864517842136E-15, 1.692578276882434470E-16 ) ) ;
#9849=ORIENTED_EDGE ( 'NONE', *, *, #13282, .T. ) ;
#9854=VERTEX_POINT ( 'NONE', #16598 ) ;
#9858=EDGE_CURVE ( 'NONE', #3659, #14934, #3786, .T. ) ;
#9864=ORIENTED_EDGE ( 'NONE', *, *, #7014, .F. ) ;
#9865=EDGE_CURVE ( 'NONE', #1935, #3596, #6046, .T. ) ;
#9871=DIRECTION ( 'NONE',  ( -5.204170427930409450E-16, 0.000000000000000000, 1.000000000000000000 ) ) ;
#9881=VECTOR ( 'NONE', #17759, 1000.000000000000000 ) ;
#9884=VECTOR ( 'NONE', #15510, 1000.000000000000000 ) ;
#9887=DIRECTION ( 'NONE',  ( 1.156482317317869999E-16, 0.000000000000000000, 1.000000000000000000 ) ) ;
#9890=DIRECTION ( 'NONE',  ( 0.000000000000000000, 0.000000000000000000, 1.000000000000000000 ) ) ;
#9903=CARTESIAN_POINT ( 'NONE',  ( -67.44681693414594292, 91.21279551874751235, 15.00000000000006928 ) ) ;
#9907=LINE ( 'NONE', #2802, #5075 ) ;
#9917=ORIENTED_EDGE ( 'NONE', *, *, #1830, .F. ) ;
#9919=CIRCLE ( 'NONE', #4811, 4.599999999999992539 ) ;
#9932=AXIS2_PLACEMENT_3D ( 'NONE', #10624, #13339, #4806 ) ;
#9934=CARTESIAN_POINT ( 'NONE',  ( -45.39578445746348478, 88.67024416760654049, -15.00000000000001421 ) ) ;
#9940=CARTESIAN_POINT ( 'NONE',  ( -48.21445538031289857, 89.37090336996882911, 15.00000000000006928 ) ) ;
#9945=CIRCLE ( 'NONE', #5139, 10.24900000000001477 ) ;
#9947=CARTESIAN_POINT ( 'NONE',  ( -57.08002265617300708, 84.22855780814606419, 15.00000000000006928 ) ) ;
#9948=VERTEX_POINT ( 'NONE', #10369 ) ;
#9950=ORIENTED_EDGE ( 'NONE', *, *, #14954, .F. ) ;
#9966=VECTOR ( 'NONE', #8003, 1000.000000000000000 ) ;
#9968=CARTESIAN_POINT ( 'NONE',  ( -57.08002265617300708, 84.22855780814606419, -15.00000000000001421 ) ) ;
#9979=ORIENTED_EDGE ( 'NONE', *, *, #7113, .T. ) ;
#9982=EDGE_LOOP ( 'NONE', ( #6792, #14238, #17918, #50 ) ) ;
#9986=ORIENTED_EDGE ( 'NONE', *, *, #13675, .F. ) ;
#9994=ORIENTED_EDGE ( 'NONE', *, *, #11467, .T. ) ;
#10001=DIRECTION ( 'NONE',  ( 0.000000000000000000, 0.000000000000000000, 1.000000000000000000 ) ) ;
#10005=AXIS2_PLACEMENT_3D ( 'NONE', #17869, #3476, #16287 ) ;
#10017=CIRCLE ( 'NONE', #9095, 4.599999999999999645 ) ;
#10018=DIRECTION ( 'NONE',  ( 0.000000000000000000, 0.000000000000000000, 1.000000000000000000 ) ) ;
#10019=( NAMED_UNIT ( * ) PLANE_ANGLE_UNIT ( ) SI_UNIT ( $, .RADIAN. ) );
#10033=DIRECTION ( 'NONE',  ( 0.000000000000000000, 0.000000000000000000, 1.000000000000000000 ) ) ;
#10035=FACE_OUTER_BOUND ( 'NONE', #12679, .T. ) ;
#10037=EDGE_CURVE ( 'NONE', #15366, #14959, #2477, .T. ) ;
#10038=DIRECTION ( 'NONE',  ( -5.204170427930409450E-16, 0.000000000000000000, 1.000000000000000000 ) ) ;
#10045=DIRECTION ( 'NONE',  ( 0.000000000000000000, 0.000000000000000000, 1.000000000000000000 ) ) ;
#10054=CARTESIAN_POINT ( 'NONE',  ( -68.76426085488260753, 88.67024416760638417, -167.1454815528550739 ) ) ;
#10076=CARTESIAN_POINT ( 'NONE',  ( -54.80923614058017534, 94.79374675277698259, -15.00000000000001421 ) ) ;
#10077=ORIENTED_EDGE ( 'NONE', *, *, #12838, .T. ) ;
#10085=EDGE_CURVE ( 'NONE', #13750, #15130, #5157, .T. ) ;
#10086=DIRECTION ( 'NONE',  ( 0.000000000000000000, 0.000000000000000000, 1.000000000000000000 ) ) ;
#10089=ORIENTED_EDGE ( 'NONE', *, *, #1982, .T. ) ;
#10099=DIRECTION ( 'NONE',  ( -1.000000000000000000, 0.000000000000000000, 0.000000000000000000 ) ) ;
#10110=ORIENTED_EDGE ( 'NONE', *, *, #16258, .F. ) ;
#10122=DIRECTION ( 'NONE',  ( -5.204170427930409450E-16, 0.000000000000000000, 1.000000000000000000 ) ) ;
#10126=VERTEX_POINT ( 'NONE', #13228 ) ;
#10127=EDGE_CURVE ( 'NONE', #2450, #2040, #12948, .T. ) ;
#10129=DIRECTION ( 'NONE',  ( -5.204170427930409450E-16, 0.000000000000000000, 1.000000000000000000 ) ) ;
#10135=EDGE_CURVE ( 'NONE', #1935, #11356, #15637, .T. ) ;
#10148=DIRECTION ( 'NONE',  ( 1.000000000000000000, 0.000000000000000000, 0.000000000000000000 ) ) ;
#10156=EDGE_CURVE ( 'NONE', #7359, #11134, #7249, .T. ) ;
#10157=DIRECTION ( 'NONE',  ( 1.156482317317869999E-16, 0.000000000000000000, 1.000000000000000000 ) ) ;
#10165=AXIS2_PLACEMENT_3D ( 'NONE', #7737, #13451, #3080 ) ;
#10171=LINE ( 'NONE', #7189, #3087 ) ;
#10174=DIRECTION ( 'NONE',  ( 1.156482317317869999E-16, 0.000000000000000000, 1.000000000000000000 ) ) ;
#10179=EDGE_CURVE ( 'NONE', #2688, #17079, #15007, .T. ) ;
#10186=CARTESIAN_POINT ( 'NONE',  ( -65.16279959635889441, 77.92691374209478283, -15.00000000000001243 ) ) ;
#10199=CIRCLE ( 'NONE', #2126, 12.49999999999999112 ) ;
#10200=CIRCLE ( 'NONE', #6594, 4.600000000000006750 ) ;
#10209=CIRCLE ( 'NONE', #13788, 4.600000000000006750 ) ;
#10211=CARTESIAN_POINT ( 'NONE',  ( -53.29103256796045684, 73.45256821284057480, -167.1454815528550739 ) ) ;
#10224=VERTEX_POINT ( 'NONE', #13059 ) ;
#10228=CARTESIAN_POINT ( 'NONE',  ( -50.90853507983961634, 93.09943318379598054, 15.00000000000006928 ) ) ;
#10243=AXIS2_PLACEMENT_3D ( 'NONE', #16288, #572, #855 ) ;
#10244=EDGE_LOOP ( 'NONE', ( #3717, #10438, #5556, #10110 ) ) ;
#10249=ORIENTED_EDGE ( 'NONE', *, *, #3325, .T. ) ;
#10250=DIRECTION ( 'NONE',  ( -5.204170427930409450E-16, 0.000000000000000000, 1.000000000000000000 ) ) ;
#10258=DIRECTION ( 'NONE',  ( 1.000000000000000000, 0.000000000000000000, 0.000000000000000000 ) ) ;
#10261=VERTEX_POINT ( 'NONE', #14537 ) ;
#10274=CYLINDRICAL_SURFACE ( 'NONE', #4212, 4.600000000000006750 ) ;
#10277=CYLINDRICAL_SURFACE ( 'NONE', #7244, 4.599999999999992539 ) ;
#10282=DIRECTION ( 'NONE',  ( 0.000000000000000000, 0.000000000000000000, 1.000000000000000000 ) ) ;
#10285=ORIENTED_EDGE ( 'NONE', *, *, #18438, .T. ) ;
#10290=AXIS2_PLACEMENT_3D ( 'NONE', #5973, #6339, #16073 ) ;
#10312=CARTESIAN_POINT ( 'NONE',  ( -65.41598826576338865, 91.10542963993673027, -15.00000000000001421 ) ) ;
#10322=CARTESIAN_POINT ( 'NONE',  ( -57.08002265617300708, 84.22855780814606419, -15.00000000000001421 ) ) ;
#10331=DIRECTION ( 'NONE',  ( -1.000000000000000000, 0.000000000000000000, 1.387778780781446662E-16 ) ) ;
#10335=EDGE_CURVE ( 'NONE', #703, #2929, #13821, .T. ) ;
#10342=DIRECTION ( 'NONE',  ( 0.000000000000000000, 0.000000000000000000, 1.000000000000000000 ) ) ;
#10343=ORIENTED_EDGE ( 'NONE', *, *, #17806, .F. ) ;
#10345=CARTESIAN_POINT ( 'NONE',  ( -66.96222586426215173, 88.60139997190893268, -167.1454815528550739 ) ) ;
#10347=VERTEX_POINT ( 'NONE', #13972 ) ;
#10357=CARTESIAN_POINT ( 'NONE',  ( -46.36441787118067026, 82.83016482797245317, -167.1454815528550739 ) ) ;
#10359=ORIENTED_EDGE ( 'NONE', *, *, #4814, .T. ) ;
#10361=CYLINDRICAL_SURFACE ( 'NONE', #5227, 4.599999999999999645 ) ;
#10369=CARTESIAN_POINT ( 'NONE',  ( -58.51182448057780050, 96.64628479562776420, -15.00000000000001421 ) ) ;
#10370=DIRECTION ( 'NONE',  ( -1.000000000000000000, 6.550315845288414753E-14, 1.387778780781443703E-16 ) ) ;
#10386=CARTESIAN_POINT ( 'NONE',  ( -59.35080917176598092, 94.79374675277695417, 15.00000000000006928 ) ) ;
#10391=VERTEX_POINT ( 'NONE', #12851 ) ;
#10392=CARTESIAN_POINT ( 'NONE',  ( -57.08002265617300708, 84.22855780814606419, -167.1454815528550739 ) ) ;
#10397=ORIENTED_EDGE ( 'NONE', *, *, #1820, .F. ) ;
#10398=EDGE_CURVE ( 'NONE', #9366, #14319, #18320, .T. ) ;
#10412=ORIENTED_EDGE ( 'NONE', *, *, #2178, .F. ) ;
#10419=ORIENTED_EDGE ( 'NONE', *, *, #309, .F. ) ;
#10424=VERTEX_POINT ( 'NONE', #18270 ) ;
#10429=EDGE_CURVE ( 'NONE', #15321, #12181, #1349, .T. ) ;
#10438=ORIENTED_EDGE ( 'NONE', *, *, #10179, .T. ) ;
#10442=CARTESIAN_POINT ( 'NONE',  ( -57.08002265617300708, 84.22855780814606419, 15.00000000000006928 ) ) ;
#10448=CARTESIAN_POINT ( 'NONE',  ( -57.08002265617300708, 84.22855780814606419, -15.00000000000001421 ) ) ;
#10451=DIRECTION ( 'NONE',  ( 1.156482317317869999E-16, 0.000000000000000000, 1.000000000000000000 ) ) ;
#10454=VERTEX_POINT ( 'NONE', #16859 ) ;
#10455=DIRECTION ( 'NONE',  ( 1.000000000000000000, 0.000000000000000000, 5.551115123125780730E-16 ) ) ;
#10457=ORIENTED_EDGE ( 'NONE', *, *, #14970, .F. ) ;
#10458=DIRECTION ( 'NONE',  ( 1.000000000000000000, 0.000000000000000000, 3.771137991253928573E-16 ) ) ;
#10468=DIRECTION ( 'NONE',  ( 0.000000000000000000, 0.000000000000000000, 1.000000000000000000 ) ) ;
#10470=AXIS2_PLACEMENT_3D ( 'NONE', #5011, #9428, #13444 ) ;
#10479=FACE_OUTER_BOUND ( 'NONE', #6747, .T. ) ;
#10480=CARTESIAN_POINT ( 'NONE',  ( -67.50540723371459251, 87.07303407725210320, -167.1454815528550739 ) ) ;
#10481=EDGE_LOOP ( 'NONE', ( #7078, #1903, #1768, #1234 ) ) ;
#10482=AXIS2_PLACEMENT_3D ( 'NONE', #3031, #3128, #42 ) ;
#10490=CIRCLE ( 'NONE', #2135, 4.599999999999992539 ) ;
#10498=ORIENTED_EDGE ( 'NONE', *, *, #4337, .F. ) ;
#10515=CARTESIAN_POINT ( 'NONE',  ( -46.10942163047475617, 78.23723799236688592, -15.00000000000001421 ) ) ;
#10519=ORIENTED_EDGE ( 'NONE', *, *, #5828, .T. ) ;
#10521=CARTESIAN_POINT ( 'NONE',  ( -46.38449965345759551, 85.77305660501679085, -167.1454815528550739 ) ) ;
#10537=DIRECTION ( 'NONE',  ( 0.000000000000000000, 0.000000000000000000, 1.000000000000000000 ) ) ;
#10540=VECTOR ( 'NONE', #17824, 1000.000000000000000 ) ;
#10544=AXIS2_PLACEMENT_3D ( 'NONE', #10442, #4645, #179 ) ;
#10546=LINE ( 'NONE', #6218, #17164 ) ;
#10547=VERTEX_POINT ( 'NONE', #7227 ) ;
#10552=DIRECTION ( 'NONE',  ( 0.000000000000000000, 0.000000000000000000, 1.000000000000000000 ) ) ;
#10573=DIRECTION ( 'NONE',  ( 0.000000000000000000, 0.000000000000000000, 1.000000000000000000 ) ) ;
#10583=DIRECTION ( 'NONE',  ( 0.000000000000000000, 0.000000000000000000, 1.000000000000000000 ) ) ;
#10584=ORIENTED_EDGE ( 'NONE', *, *, #15902, .T. ) ;
#10585=VECTOR ( 'NONE', #3880, 1000.000000000000000 ) ;
#10587=AXIS2_PLACEMENT_3D ( 'NONE', #16593, #601, #3583 ) ;
#10590=CARTESIAN_POINT ( 'NONE',  ( -57.08002265617300708, 84.22855780814606419, -167.1454815528550739 ) ) ;
#10591=DIRECTION ( 'NONE',  ( 1.000000000000000000, 0.000000000000000000, 5.077734830647299712E-16 ) ) ;
#10593=EDGE_CURVE ( 'NONE', #11848, #15321, #12042, .T. ) ;
#10596=ORIENTED_EDGE ( 'NONE', *, *, #15319, .F. ) ;
#10597=DIRECTION ( 'NONE',  ( 1.000000000000000000, 0.000000000000000000, 3.771137991253928573E-16 ) ) ;
#10600=VECTOR ( 'NONE', #14643, 1000.000000000000000 ) ;
#10603=LINE ( 'NONE', #11904, #11501 ) ;
#10607=DIRECTION ( 'NONE',  ( 1.000000000000000000, 0.000000000000000000, 5.551115123125777772E-16 ) ) ;
#10611=VERTEX_POINT ( 'NONE', #3271 ) ;
#10616=CARTESIAN_POINT ( 'NONE',  ( -63.34052343625892689, 73.40930968350525632, -167.1454815528550739 ) ) ;
#10617=ORIENTED_EDGE ( 'NONE', *, *, #18455, .T. ) ;
#10623=ORIENTED_EDGE ( 'NONE', *, *, #17697, .T. ) ;
#10624=CARTESIAN_POINT ( 'NONE',  ( -57.89103256796045116, 73.45256821284057480, -167.1454815528550739 ) ) ;
#10643=CYLINDRICAL_SURFACE ( 'NONE', #13865, 12.50000000000001066 ) ;
#10646=FACE_OUTER_BOUND ( 'NONE', #16229, .T. ) ;
#10669=CYLINDRICAL_SURFACE ( 'NONE', #7044, 12.49999999999999645 ) ;
#10678=CARTESIAN_POINT ( 'NONE',  ( -57.08002265617300708, 84.22855780814606419, -15.00000000000001421 ) ) ;
#10691=VERTEX_POINT ( 'NONE', #11881 ) ;
#10701=DIRECTION ( 'NONE',  ( -1.000000000000000000, 0.000000000000000000, 1.692578276882434470E-16 ) ) ;
#10709=VECTOR ( 'NONE', #17215, 1000.000000000000000 ) ;
#10714=DIRECTION ( 'NONE',  ( 1.000000000000000000, 0.000000000000000000, 3.771137991253923150E-16 ) ) ;
#10720=CARTESIAN_POINT ( 'NONE',  ( -64.75543355702687620, 94.09456345901884333, -167.1454815528550739 ) ) ;
#10722=CYLINDRICAL_SURFACE ( 'NONE', #719, 12.50000000000001066 ) ;
#10724=LINE ( 'NONE', #16243, #16738 ) ;
#10725=CARTESIAN_POINT ( 'NONE',  ( -46.95762973216378811, 85.83453492254348305, -15.00000000000001421 ) ) ;
#10726=DIRECTION ( 'NONE',  ( 1.000000000000000000, 0.000000000000000000, 0.000000000000000000 ) ) ;
#10727=FACE_OUTER_BOUND ( 'NONE', #8842, .T. ) ;
#10731=EDGE_CURVE ( 'NONE', #14319, #9948, #7569, .T. ) ;
#10732=ORIENTED_EDGE ( 'NONE', *, *, #10085, .F. ) ;
#10741=EDGE_CURVE ( 'NONE', #415, #9366, #11459, .T. ) ;
#10743=EDGE_CURVE ( 'NONE', #11134, #16609, #1880, .T. ) ;
#10744=DIRECTION ( 'NONE',  ( 1.000000000000000000, 0.000000000000000000, 3.771137991253934490E-16 ) ) ;
#10746=CARTESIAN_POINT ( 'NONE',  ( -68.05062368187118693, 78.23723799236674381, -167.1454815528550739 ) ) ;
#10747=CARTESIAN_POINT ( 'NONE',  ( -49.93060289285580922, 91.57211267264388255, -15.00000000000001421 ) ) ;
#10761=ORIENTED_EDGE ( 'NONE', *, *, #17502, .F. ) ;
#10762=EDGE_CURVE ( 'NONE', #7723, #13519, #9053, .T. ) ;
#10764=CIRCLE ( 'NONE', #10165, 12.49999999999999112 ) ;
#10782=ORIENTED_EDGE ( 'NONE', *, *, #10398, .T. ) ;
#10785=AXIS2_PLACEMENT_3D ( 'NONE', #17810, #14818, #4990 ) ;
#10802=EDGE_CURVE ( 'NONE', #14319, #12661, #13434, .T. ) ;
#10804=DIRECTION ( 'NONE',  ( 1.000000000000000000, 0.000000000000000000, 0.000000000000000000 ) ) ;
#10806=AXIS2_PLACEMENT_3D ( 'NONE', #114, #16, #11613 ) ;
#10807=DIRECTION ( 'NONE',  ( 1.000000000000000000, 0.000000000000000000, 5.551115123125777772E-16 ) ) ;
#10816=ORIENTED_EDGE ( 'NONE', *, *, #539, .T. ) ;
#10819=CARTESIAN_POINT ( 'NONE',  ( -67.77554565888843285, 85.77305660501664875, -167.1454815528550739 ) ) ;
#10822=CARTESIAN_POINT ( 'NONE',  ( -48.43547250063686960, 78.72276507608465579, 15.00000000000009592 ) ) ;
#10823=CIRCLE ( 'NONE', #3349, 10.24900000000000766 ) ;
#10825=CARTESIAN_POINT ( 'NONE',  ( -56.41614838398844256, 95.01461175692088545, 15.00000000000006928 ) ) ;
#10826=DIRECTION ( 'NONE',  ( 1.000000000000000000, 0.000000000000000000, 3.771137991253928573E-16 ) ) ;
#10831=VECTOR ( 'NONE', #9208, 1000.000000000000000 ) ;
#10837=AXIS2_PLACEMENT_3D ( 'NONE', #15816, #1598, #16071 ) ;
#10839=CARTESIAN_POINT ( 'NONE',  ( -48.43547250063686960, 78.72276507608465579, -15.00000000000001421 ) ) ;
#10841=DIRECTION ( 'NONE',  ( 1.156482317317869999E-16, 0.000000000000000000, 1.000000000000000000 ) ) ;
#10844=EDGE_CURVE ( 'NONE', #10849, #18394, #13712, .T. ) ;
#10846=CARTESIAN_POINT ( 'NONE',  ( -58.51182448057780050, 96.64628479562776420, 15.00000000000006928 ) ) ;
#10849=VERTEX_POINT ( 'NONE', #3422 ) ;
#10852=AXIS2_PLACEMENT_3D ( 'NONE', #8901, #5813, #17227 ) ;
#10853=VECTOR ( 'NONE', #8782, 1000.000000000000000 ) ;
#10855=ORIENTED_EDGE ( 'NONE', *, *, #7357, .F. ) ;
#10856=EDGE_CURVE ( 'NONE', #14316, #6278, #7269, .T. ) ;
#10866=DIRECTION ( 'NONE',  ( -5.204170427930409450E-16, 0.000000000000000000, 1.000000000000000000 ) ) ;
#10878=ORIENTED_EDGE ( 'NONE', *, *, #1563, .F. ) ;
#10885=AXIS2_PLACEMENT_3D ( 'NONE', #10819, #3515, #10928 ) ;
#10887=DIRECTION ( 'NONE',  ( 1.000000000000000000, 0.000000000000000000, 0.000000000000000000 ) ) ;
#10890=PRODUCT_DEFINITION_SHAPE ( 'NONE', 'NONE',  #13786 ) ;
#10895=CARTESIAN_POINT ( 'NONE',  ( -65.72457281170906640, 78.72276507608454210, 15.00000000000006928 ) ) ;
#10900=EDGE_CURVE ( 'NONE', #2011, #10849, #11174, .T. ) ;
#10906=CARTESIAN_POINT ( 'NONE',  ( -57.08002265617300708, 84.22855780814606419, 15.00000000000006928 ) ) ;
#10908=CARTESIAN_POINT ( 'NONE',  ( -62.11705611183893438, 93.78931001713317528, -167.1454815528550739 ) ) ;
#10913=CARTESIAN_POINT ( 'NONE',  ( -57.08002265617300708, 84.22855780814606419, 15.00000000000006928 ) ) ;
#10916=AXIS2_PLACEMENT_3D ( 'NONE', #13748, #7950, #2242 ) ;
#10928=DIRECTION ( 'NONE',  ( 1.000000000000000000, 0.000000000000000000, 0.000000000000000000 ) ) ;
#10930=CARTESIAN_POINT ( 'NONE',  ( -67.20241558018224737, 85.83453492254335515, -15.00000000000001243 ) ) ;
#10944=DIRECTION ( 'NONE',  ( 0.000000000000000000, 0.000000000000000000, 1.000000000000000000 ) ) ;
#10946=ORIENTED_EDGE ( 'NONE', *, *, #11765, .T. ) ;
#10952=FACE_OUTER_BOUND ( 'NONE', #17678, .T. ) ;
#10956=ORIENTED_EDGE ( 'NONE', *, *, #17950, .T. ) ;
#10959=ORIENTED_EDGE ( 'NONE', *, *, #3791, .F. ) ;
#10962=PRODUCT_DEFINITION_CONTEXT ( 'detailed design', #12931, 'design' ) ;
#10974=ORIENTED_EDGE ( 'NONE', *, *, #4814, .F. ) ;
#10992=FACE_OUTER_BOUND ( 'NONE', #11580, .T. ) ;
#10995=VERTEX_POINT ( 'NONE', #13915 ) ;
#11000=CARTESIAN_POINT ( 'NONE',  ( -57.08002265617300708, 84.22855780814606419, 15.00000000000006928 ) ) ;
#11021=DIRECTION ( 'NONE',  ( 1.000000000000000000, 0.000000000000000000, 0.000000000000000000 ) ) ;
#11022=CARTESIAN_POINT ( 'NONE',  ( -57.08002265617300708, 84.22855780814606419, -167.1454815528550739 ) ) ;
#11033=DIRECTION ( 'NONE',  ( 0.000000000000000000, 0.000000000000000000, 1.000000000000000000 ) ) ;
#11041=ORIENTED_EDGE ( 'NONE', *, *, #548, .F. ) ;
#11054=CIRCLE ( 'NONE', #4476, 4.600000000000006750 ) ;
#11055=DIRECTION ( 'NONE',  ( 1.156482317317869999E-16, 0.000000000000000000, 1.000000000000000000 ) ) ;
#11065=VERTEX_POINT ( 'NONE', #5756 ) ;
#11076=CARTESIAN_POINT ( 'NONE',  ( -57.08002265617300708, 84.22855780814606419, 15.00000000000006928 ) ) ;
#11077=ORIENTED_EDGE ( 'NONE', *, *, #4797, .T. ) ;
#11082=ADVANCED_FACE ( 'NONE', ( #11485 ), #3303, .T. ) ;
#11088=CARTESIAN_POINT ( 'NONE',  ( -63.37199650155329778, 75.44273092821040905, -15.00000000000001421 ) ) ;
#11091=DIRECTION ( 'NONE',  ( -5.204170427930409450E-16, 0.000000000000000000, 1.000000000000000000 ) ) ;
#11103=CYLINDRICAL_SURFACE ( 'NONE', #4314, 4.599999999999999645 ) ;
#11108=CARTESIAN_POINT ( 'NONE',  ( -61.98305514952129158, 93.22868410554717400, -167.1454815528550739 ) ) ;
#11122=ORIENTED_EDGE ( 'NONE', *, *, #297, .T. ) ;
#11127=ADVANCED_FACE ( 'NONE', ( #15855 ), #14627, .T. ) ;
#11128=CYLINDRICAL_SURFACE ( 'NONE', #2412, 4.599999999999992539 ) ;
#11134=VERTEX_POINT ( 'NONE', #8933 ) ;
#11149=DIRECTION ( 'NONE',  ( 0.000000000000000000, 0.000000000000000000, 1.000000000000000000 ) ) ;
#11150=AXIS2_PLACEMENT_3D ( 'NONE', #13132, #4694, #14452 ) ;
#11155=AXIS2_PLACEMENT_3D ( 'NONE', #4463, #10174, #1845 ) ;
#11158=CARTESIAN_POINT ( 'NONE',  ( -57.08002265617300708, 84.22855780814606419, -15.00000000000001421 ) ) ;
#11161=DIRECTION ( 'NONE',  ( 0.000000000000000000, 0.000000000000000000, 1.000000000000000000 ) ) ;
#11169=LINE ( 'NONE', #16860, #11377 ) ;
#11170=ORIENTED_EDGE ( 'NONE', *, *, #14847, .T. ) ;
#11174=CIRCLE ( 'NONE', #8780, 4.599999999999992539 ) ;
#11180=DIRECTION ( 'NONE',  ( -5.204170427930409450E-16, 0.000000000000000000, 1.000000000000000000 ) ) ;
#11190=DIRECTION ( 'NONE',  ( -1.000000000000000000, 0.000000000000000000, 0.000000000000000000 ) ) ;
#11195=ORIENTED_EDGE ( 'NONE', *, *, #12142, .T. ) ;
#11211=DIRECTION ( 'NONE',  ( 1.156482317317869999E-16, 0.000000000000000000, 1.000000000000000000 ) ) ;
#11212=CARTESIAN_POINT ( 'NONE',  ( -59.35080917176598092, 94.79374675277695417, -15.00000000000001421 ) ) ;
#11218=DIRECTION ( 'NONE',  ( -1.000000000000000000, -4.218847493575593591E-14, 1.387778780781445182E-16 ) ) ;
#11220=DIRECTION ( 'NONE',  ( 0.000000000000000000, 0.000000000000000000, 1.000000000000000000 ) ) ;
#11221=ORIENTED_EDGE ( 'NONE', *, *, #4048, .F. ) ;
#11228=EDGE_CURVE ( 'NONE', #10691, #703, #9446, .T. ) ;
#11231=EDGE_CURVE ( 'NONE', #10424, #9440, #15434, .T. ) ;
#11236=MECHANICAL_DESIGN_GEOMETRIC_PRESENTATION_REPRESENTATION('',(#16892),#2251);
#11248=VERTEX_POINT ( 'NONE', #13843 ) ;
#11267=CARTESIAN_POINT ( 'NONE',  ( -67.02098183716937285, 79.99098546104525553, 15.00000000000006928 ) ) ;
#11271=DIRECTION ( 'NONE',  ( -5.204170427930409450E-16, 0.000000000000000000, 1.000000000000000000 ) ) ;
#11275=VERTEX_POINT ( 'NONE', #16632 ) ;
#11276=DIRECTION ( 'NONE',  ( -1.000000000000000000, 0.000000000000000000, 0.000000000000000000 ) ) ;
#11280=EDGE_LOOP ( 'NONE', ( #5953, #200, #5413, #13530 ) ) ;
#11283=ORIENTED_EDGE ( 'NONE', *, *, #17501, .T. ) ;
#11289=LINE ( 'NONE', #13801, #1298 ) ;
#11317=CARTESIAN_POINT ( 'NONE',  ( -47.19781944808393348, 88.60139997190906058, -15.00000000000001421 ) ) ;
#11332=CARTESIAN_POINT ( 'NONE',  ( -51.81614838398844824, 95.01461175692088545, -167.1454815528550739 ) ) ;
#11333=LINE ( 'NONE', #11527, #10709 ) ;
#11335=AXIS2_PLACEMENT_3D ( 'NONE', #8041, #1229, #12264 ) ;
#11338=ADVANCED_FACE ( 'NONE', ( #8523, #17281 ), #4465, .T. ) ;
#11345=CARTESIAN_POINT ( 'NONE',  ( -67.88623620617454435, 84.15481808402788033, -15.00000000000001421 ) ) ;
#11347=VECTOR ( 'NONE', #5101, 1000.000000000000000 ) ;
#11356=VERTEX_POINT ( 'NONE', #1320 ) ;
#11363=DIRECTION ( 'NONE',  ( 1.156482317317869999E-16, 0.000000000000000000, 1.000000000000000000 ) ) ;
#11374=DIRECTION ( 'NONE',  ( -5.204170427930409450E-16, 0.000000000000000000, 1.000000000000000000 ) ) ;
#11377=VECTOR ( 'NONE', #6563, 1000.000000000000000 ) ;
#11402=VECTOR ( 'NONE', #16675, 1000.000000000000000 ) ;
#11413=AXIS2_PLACEMENT_3D ( 'NONE', #7224, #3014, #8724 ) ;
#11419=AXIS2_PLACEMENT_3D ( 'NONE', #9011, #3667, #11903 ) ;
#11423=LINE ( 'NONE', #7968, #5724 ) ;
#11426=AXIS2_PLACEMENT_3D ( 'NONE', #10521, #2103, #10804 ) ;
#11435=CARTESIAN_POINT ( 'NONE',  ( -66.88945454405379110, 81.25920652595873150, -15.00000000000001421 ) ) ;
#11438=CIRCLE ( 'NONE', #3651, 12.49999999999999112 ) ;
#11444=EDGE_CURVE ( 'NONE', #848, #4970, #4825, .T. ) ;
#11446=CIRCLE ( 'NONE', #974, 4.600000000000006750 ) ;
#11448=DIRECTION ( 'NONE',  ( 0.000000000000000000, 0.000000000000000000, 1.000000000000000000 ) ) ;
#11450=EDGE_CURVE ( 'NONE', #6999, #3974, #10546, .T. ) ;
#11456=ORIENTED_EDGE ( 'NONE', *, *, #150, .F. ) ;
#11459=CIRCLE ( 'NONE', #16205, 4.599999999999999645 ) ;
#11460=CARTESIAN_POINT ( 'NONE',  ( -68.76426085488260753, 88.67024416760638417, -15.00000000000001421 ) ) ;
#11463=ORIENTED_EDGE ( 'NONE', *, *, #8374, .T. ) ;
#11467=EDGE_CURVE ( 'NONE', #6109, #16861, #5790, .T. ) ;
#11469=DIRECTION ( 'NONE',  ( 1.156482317317869999E-16, 0.000000000000000000, 1.000000000000000000 ) ) ;
#11470=DIRECTION ( 'NONE',  ( 1.000000000000000000, 0.000000000000000000, 5.077734830647302671E-16 ) ) ;
#11473=EDGE_CURVE ( 'NONE', #845, #12461, #2511, .T. ) ;
#11483=ADVANCED_FACE ( 'NONE', ( #13265 ), #7728, .T. ) ;
#11485=FACE_OUTER_BOUND ( 'NONE', #3649, .T. ) ;
#11487=AXIS2_PLACEMENT_3D ( 'NONE', #14231, #14034, #4203 ) ;
#11489=CARTESIAN_POINT ( 'NONE',  ( -60.18936887439735273, 72.12145385653096241, -167.1454815528550739 ) ) ;
#11492=ORIENTED_EDGE ( 'NONE', *, *, #5165, .T. ) ;
#11493=DIRECTION ( 'NONE',  ( -1.000000000000000000, 6.328271240363383445E-14, 1.387778780781443703E-16 ) ) ;
#11496=ORIENTED_EDGE ( 'NONE', *, *, #8346, .F. ) ;
#11501=VECTOR ( 'NONE', #13498, 1000.000000000000000 ) ;
#11507=EDGE_CURVE ( 'NONE', #9564, #16963, #6129, .T. ) ;
#11511=DIRECTION ( 'NONE',  ( 1.000000000000000000, 0.000000000000000000, 0.000000000000000000 ) ) ;
#11514=ORIENTED_EDGE ( 'NONE', *, *, #809, .T. ) ;
#11519=AXIS2_PLACEMENT_3D ( 'NONE', #16537, #648, #3457 ) ;
#11527=CARTESIAN_POINT ( 'NONE',  ( -60.71399380653853228, 72.26844686893187486, -167.1454815528550739 ) ) ;
#11531=ADVANCED_FACE ( 'NONE', ( #14920 ), #728, .T. ) ;
#11535=LINE ( 'NONE', #8718, #18512 ) ;
#11536=CARTESIAN_POINT ( 'NONE',  ( -47.15582643534892782, 86.78830982163900387, -167.1454815528550739 ) ) ;
#11538=VERTEX_POINT ( 'NONE', #16518 ) ;
#11542=AXIS2_PLACEMENT_3D ( 'NONE', #13446, #6045, #5957 ) ;
#11550=DIRECTION ( 'NONE',  ( 0.000000000000000000, 0.000000000000000000, 1.000000000000000000 ) ) ;
#11552=VERTEX_POINT ( 'NONE', #2392 ) ;
#11568=CARTESIAN_POINT ( 'NONE',  ( -46.69442755757756203, 81.24207102880484399, -167.1454815528550739 ) ) ;
#11578=CARTESIAN_POINT ( 'NONE',  ( -66.39376235201207521, 88.50596986196454452, 15.00000000000006928 ) ) ;
#11580=EDGE_LOOP ( 'NONE', ( #14047, #12886, #8589, #4651 ) ) ;
#11581=ADVANCED_FACE ( 'NONE', ( #6707 ), #10643, .T. ) ;
#11595=CARTESIAN_POINT ( 'NONE',  ( -46.95762973216378811, 85.83453492254348305, 15.00000000000006928 ) ) ;
#11597=ORIENTED_EDGE ( 'NONE', *, *, #7030, .F. ) ;
#11598=CARTESIAN_POINT ( 'NONE',  ( -60.71399380653853228, 72.26844686893187486, -15.00000000000001421 ) ) ;
#11601=CARTESIAN_POINT ( 'NONE',  ( -57.56709772515574031, 94.46597735006069740, -15.00000000000001421 ) ) ;
#11613=DIRECTION ( 'NONE',  ( 1.000000000000000000, 0.000000000000000000, 5.551115123125780730E-16 ) ) ;
#11617=ORIENTED_EDGE ( 'NONE', *, *, #4474, .T. ) ;
#11626=ORIENTED_EDGE ( 'NONE', *, *, #13840, .F. ) ;
#11627=ORIENTED_EDGE ( 'NONE', *, *, #3196, .T. ) ;
#11635=ADVANCED_FACE ( 'NONE', ( #12222 ), #10722, .T. ) ;
#11638=VECTOR ( 'NONE', #3146, 1000.000000000000000 ) ;
#11645=LINE ( 'NONE', #4528, #13139 ) ;
#11650=ORIENTED_EDGE ( 'NONE', *, *, #6165, .T. ) ;
#11653=DIRECTION ( 'NONE',  ( -5.204170427930409450E-16, 0.000000000000000000, 1.000000000000000000 ) ) ;
#11658=CYLINDRICAL_SURFACE ( 'NONE', #18386, 4.599999999999999645 ) ;
#11666=VECTOR ( 'NONE', #11149, 1000.000000000000000 ) ;
#11670=VERTEX_POINT ( 'NONE', #8299 ) ;
#11673=DIRECTION ( 'NONE',  ( -5.204170427930409450E-16, 0.000000000000000000, 1.000000000000000000 ) ) ;
#11680=CYLINDRICAL_SURFACE ( 'NONE', #6744, 10.24899999999999345 ) ;
#11684=EDGE_CURVE ( 'NONE', #18359, #6999, #3708, .T. ) ;
#11691=CARTESIAN_POINT ( 'NONE',  ( -57.08002265617300708, 84.22855780814606419, -15.00000000000001421 ) ) ;
#11699=DIRECTION ( 'NONE',  ( 1.156482317317869999E-16, 0.000000000000000000, 1.000000000000000000 ) ) ;
#11701=EDGE_CURVE ( 'NONE', #3784, #10995, #10017, .T. ) ;
#11702=CARTESIAN_POINT ( 'NONE',  ( -66.27474722583565381, 78.55081803573735044, 15.00000000000006928 ) ) ;
#11706=ORIENTED_EDGE ( 'NONE', *, *, #10593, .F. ) ;
#11708=CIRCLE ( 'NONE', #644, 10.24900000000000055 ) ;
#11711=VERTEX_POINT ( 'NONE', #14108 ) ;
#11712=AXIS2_PLACEMENT_3D ( 'NONE', #7606, #13226, #6270 ) ;
#11723=CIRCLE ( 'NONE', #12318, 10.24900000000000055 ) ;
#11730=FACE_OUTER_BOUND ( 'NONE', #3252, .T. ) ;
#11735=EDGE_CURVE ( 'NONE', #1399, #10391, #434, .T. ) ;
#11736=AXIS2_PLACEMENT_3D ( 'NONE', #955, #12762, #5624 ) ;
#11737=VECTOR ( 'NONE', #1451, 1000.000000000000000 ) ;
#11751=CIRCLE ( 'NONE', #4860, 4.600000000000006750 ) ;
#11753=DIRECTION ( 'NONE',  ( -1.000000000000000000, 0.000000000000000000, 0.000000000000000000 ) ) ;
#11758=EDGE_LOOP ( 'NONE', ( #7601, #2905, #4294, #9864 ) ) ;
#11764=ORIENTED_EDGE ( 'NONE', *, *, #6616, .F. ) ;
#11765=EDGE_CURVE ( 'NONE', #5674, #9250, #1035, .T. ) ;
#11772=CARTESIAN_POINT ( 'NONE',  ( -69.26024277767963611, 81.41924511788803898, 15.00000000000006928 ) ) ;
#11776=CIRCLE ( 'NONE', #6698, 12.50000000000001776 ) ;
#11777=CARTESIAN_POINT ( 'NONE',  ( -57.08002265617300708, 84.22855780814606419, 15.00000000000006928 ) ) ;
#11779=ORIENTED_EDGE ( 'NONE', *, *, #4452, .F. ) ;
#11782=CARTESIAN_POINT ( 'NONE',  ( -57.08002265617300708, 84.22855780814606419, -15.00000000000001421 ) ) ;
#11785=CIRCLE ( 'NONE', #8519, 4.600000000000006750 ) ;
#11790=CIRCLE ( 'NONE', #13289, 4.599999999999992539 ) ;
#11819=DIRECTION ( 'NONE',  ( -5.204170427930409450E-16, 0.000000000000000000, 1.000000000000000000 ) ) ;
#11833=VERTEX_POINT ( 'NONE', #3403 ) ;
#11839=DIRECTION ( 'NONE',  ( 1.156482317317869999E-16, 0.000000000000000000, 1.000000000000000000 ) ) ;
#11840=ORIENTED_EDGE ( 'NONE', *, *, #6432, .T. ) ;
#11846=CARTESIAN_POINT ( 'NONE',  ( -50.78804881079258848, 75.44273092821050852, -167.1454815528550739 ) ) ;
#11847=LINE ( 'NONE', #17535, #7161 ) ;
#11848=VERTEX_POINT ( 'NONE', #10515 ) ;
#11851=CARTESIAN_POINT ( 'NONE',  ( -47.76080550507955280, 75.89776002577458769, -15.00000000000001421 ) ) ;
#11855=CARTESIAN_POINT ( 'NONE',  ( -66.88945454405379110, 81.25920652595873150, -167.1454815528550739 ) ) ;
#11878=CARTESIAN_POINT ( 'NONE',  ( -66.39923980726636898, 75.89776002577445979, 15.00000000000006928 ) ) ;
#11881=CARTESIAN_POINT ( 'NONE',  ( -68.05062368187118693, 78.23723799236674381, -15.00000000000001243 ) ) ;
#11889=AXIS2_PLACEMENT_3D ( 'NONE', #7325, #14436, #15748 ) ;
#11892=CARTESIAN_POINT ( 'NONE',  ( -57.08002265617300708, 84.22855780814606419, -167.1454815528550739 ) ) ;
#11897=EDGE_CURVE ( 'NONE', #18427, #7016, #11790, .T. ) ;
#11899=EDGE_CURVE ( 'NONE', #3150, #3299, #16864, .T. ) ;
#11901=AXIS2_PLACEMENT_3D ( 'NONE', #9266, #9184, #13575 ) ;
#11902=CARTESIAN_POINT ( 'NONE',  ( -47.88529808651028929, 78.55081803573747834, -15.00000000000001421 ) ) ;
#11903=DIRECTION ( 'NONE',  ( 1.000000000000000000, 0.000000000000000000, 0.000000000000000000 ) ) ;
#11904=CARTESIAN_POINT ( 'NONE',  ( -51.85133027979232878, 95.58244595420329404, -167.1454815528550739 ) ) ;
#11905=CARTESIAN_POINT ( 'NONE',  ( -50.78804881079258848, 75.44273092821050852, -15.00000000000001421 ) ) ;
#11908=EDGE_LOOP ( 'NONE', ( #14618, #3291, #14005, #1679 ) ) ;
#11912=ORIENTED_EDGE ( 'NONE', *, *, #7535, .F. ) ;
#11915=ORIENTED_EDGE ( 'NONE', *, *, #7014, .T. ) ;
#11928=ORIENTED_EDGE ( 'NONE', *, *, #1381, .T. ) ;
#11936=DIRECTION ( 'NONE',  ( 0.000000000000000000, 0.000000000000000000, 1.000000000000000000 ) ) ;
#11947=CARTESIAN_POINT ( 'NONE',  ( -57.08002265617300708, 84.22855780814606419, -15.00000000000001421 ) ) ;
#11960=AXIS2_PLACEMENT_3D ( 'NONE', #17100, #12501, #879 ) ;
#11965=LINE ( 'NONE', #2046, #17159 ) ;
#11967=AXIS2_PLACEMENT_3D ( 'NONE', #15704, #10250, #14635 ) ;
#11974=LINE ( 'NONE', #8902, #5962 ) ;
#11982=AXIS2_PLACEMENT_3D ( 'NONE', #16592, #3782, #10701 ) ;
#11983=VERTEX_POINT ( 'NONE', #17808 ) ;
#11985=DIRECTION ( 'NONE',  ( 1.000000000000000000, 0.000000000000000000, 4.625929269271485914E-16 ) ) ;
#11991=DIRECTION ( 'NONE',  ( -5.204170427930409450E-16, 0.000000000000000000, 1.000000000000000000 ) ) ;
#11993=ORIENTED_EDGE ( 'NONE', *, *, #16777, .F. ) ;
#12010=CIRCLE ( 'NONE', #13209, 4.599999999999999645 ) ;
#12014=EDGE_CURVE ( 'NONE', #2791, #18427, #18377, .T. ) ;
#12015=ORIENTED_EDGE ( 'NONE', *, *, #6196, .F. ) ;
#12023=CARTESIAN_POINT ( 'NONE',  ( -68.30128029835485393, 78.72098330317788850, -15.00000000000001421 ) ) ;
#12032=ORIENTED_EDGE ( 'NONE', *, *, #13485, .T. ) ;
#12035=ORIENTED_EDGE ( 'NONE', *, *, #10731, .T. ) ;
#12041=VECTOR ( 'NONE', #5315, 1000.000000000000000 ) ;
#12042=CIRCLE ( 'NONE', #10852, 12.49999999999999112 ) ;
#12046=DIRECTION ( 'NONE',  ( 1.000000000000000000, 0.000000000000000000, 3.771137991253917233E-16 ) ) ;
#12050=FACE_OUTER_BOUND ( 'NONE', #5878, .T. ) ;
#12052=ORIENTED_EDGE ( 'NONE', *, *, #3879, .T. ) ;
#12073=CYLINDRICAL_SURFACE ( 'NONE', #3935, 4.599999999999999645 ) ;
#12082=EDGE_CURVE ( 'NONE', #274, #1231, #6869, .T. ) ;
#12088=DIRECTION ( 'NONE',  ( 1.000000000000000000, 0.000000000000000000, 0.000000000000000000 ) ) ;
#12108=ORIENTED_EDGE ( 'NONE', *, *, #4360, .T. ) ;
#12118=EDGE_CURVE ( 'NONE', #70, #18394, #8527, .T. ) ;
#12120=EDGE_LOOP ( 'NONE', ( #12344, #1786, #14789, #10959 ) ) ;
#12134=ORIENTED_EDGE ( 'NONE', *, *, #12142, .F. ) ;
#12135=DIRECTION ( 'NONE',  ( -5.204170427930409450E-16, 0.000000000000000000, 1.000000000000000000 ) ) ;
#12139=CARTESIAN_POINT ( 'NONE',  ( -55.64822083176820655, 96.64628479562776420, -167.1454815528550739 ) ) ;
#12142=EDGE_CURVE ( 'NONE', #9222, #11711, #1171, .T. ) ;
#12146=CARTESIAN_POINT ( 'NONE',  ( -64.75543355702687620, 94.09456345901884333, -15.00000000000001421 ) ) ;
#12148=DIRECTION ( 'NONE',  ( 0.000000000000000000, 0.000000000000000000, 1.000000000000000000 ) ) ;
#12151=ORIENTED_EDGE ( 'NONE', *, *, #12240, .F. ) ;
#12159=ORIENTED_EDGE ( 'NONE', *, *, #15103, .T. ) ;
#12166=CARTESIAN_POINT ( 'NONE',  ( -57.08002265617300708, 84.22855780814606419, 15.00000000000006928 ) ) ;
#12173=DIRECTION ( 'NONE',  ( 1.156482317317869999E-16, 0.000000000000000000, 1.000000000000000000 ) ) ;
#12179=FACE_OUTER_BOUND ( 'NONE', #12120, .T. ) ;
#12181=VERTEX_POINT ( 'NONE', #3965 ) ;
#12182=LINE ( 'NONE', #959, #12552 ) ;
#12190=CARTESIAN_POINT ( 'NONE',  ( -57.08002265617300708, 84.22855780814606419, 15.00000000000006928 ) ) ;
#12193=ORIENTED_EDGE ( 'NONE', *, *, #828, .T. ) ;
#12198=CYLINDRICAL_SURFACE ( 'NONE', #14136, 10.24900000000001477 ) ;
#12208=FACE_OUTER_BOUND ( 'NONE', #15960, .T. ) ;
#12214=VERTEX_POINT ( 'NONE', #12782 ) ;
#12221=VECTOR ( 'NONE', #15413, 1000.000000000000000 ) ;
#12222=FACE_OUTER_BOUND ( 'NONE', #145, .T. ) ;
#12231=CARTESIAN_POINT ( 'NONE',  ( -57.08002265617300708, 84.22855780814606419, -167.1454815528550739 ) ) ;
#12237=ORIENTED_EDGE ( 'NONE', *, *, #13675, .T. ) ;
#12240=EDGE_CURVE ( 'NONE', #16069, #2011, #14785, .T. ) ;
#12245=DIRECTION ( 'NONE',  ( -1.000000000000000000, 0.000000000000000000, 1.692578276882436442E-16 ) ) ;
#12249=ADVANCED_FACE ( 'NONE', ( #9082 ), #10669, .T. ) ;
#12250=CARTESIAN_POINT ( 'NONE',  ( -57.08002265617300708, 84.22855780814606419, -167.1454815528550739 ) ) ;
#12252=CARTESIAN_POINT ( 'NONE',  ( -60.76828531927866095, 74.07097899412299569, -167.1454815528550739 ) ) ;
#12264=DIRECTION ( 'NONE',  ( -1.000000000000000000, -1.354062621505947576E-15, 1.692578276882434470E-16 ) ) ;
#12268=EDGE_CURVE ( 'NONE', #113, #10347, #8215, .T. ) ;
#12269=VECTOR ( 'NONE', #10282, 1000.000000000000000 ) ;
#12271=EDGE_LOOP ( 'NONE', ( #8548, #7184, #1120, #10855 ) ) ;
#12305=CARTESIAN_POINT ( 'NONE',  ( -50.35400969968294049, 73.69239390902568232, -167.1454815528550739 ) ) ;
#12306=DIRECTION ( 'NONE',  ( 1.000000000000000000, 0.000000000000000000, 0.000000000000000000 ) ) ;
#12318=AXIS2_PLACEMENT_3D ( 'NONE', #17287, #4470, #2988 ) ;
#12321=CARTESIAN_POINT ( 'NONE',  ( -57.08002265617300708, 84.22855780814606419, -167.1454815528550739 ) ) ;
#12327=CARTESIAN_POINT ( 'NONE',  ( -67.32681558843928826, 84.01587117655452630, -15.00000000000001421 ) ) ;
#12336=CARTESIAN_POINT ( 'NONE',  ( -54.75080917176597950, 94.79374675277695417, 15.00000000000007105 ) ) ;
#12338=DIRECTION ( 'NONE',  ( 0.000000000000000000, 0.000000000000000000, 1.000000000000000000 ) ) ;
#12341=CIRCLE ( 'NONE', #7561, 12.50000000000000355 ) ;
#12344=ORIENTED_EDGE ( 'NONE', *, *, #14873, .F. ) ;
#12348=AXIS2_PLACEMENT_3D ( 'NONE', #18153, #5322, #9225 ) ;
#12350=ORIENTED_EDGE ( 'NONE', *, *, #17270, .F. ) ;
#12358=VERTEX_POINT ( 'NONE', #16273 ) ;
#12360=ADVANCED_FACE ( 'NONE', ( #13565 ), #4029, .T. ) ;
#12369=EDGE_LOOP ( 'NONE', ( #4431, #4120, #9849, #3496 ) ) ;
#12381=ADVANCED_FACE ( 'NONE', ( #9634 ), #12544, .T. ) ;
#12396=AXIS2_PLACEMENT_3D ( 'NONE', #6085, #11819, #16742 ) ;
#12406=AXIS2_PLACEMENT_3D ( 'NONE', #9777, #6967, #4253 ) ;
#12416=DIRECTION ( 'NONE',  ( 0.000000000000000000, 0.000000000000000000, 1.000000000000000000 ) ) ;
#12418=DIRECTION ( 'NONE',  ( 0.000000000000000000, 0.000000000000000000, 1.000000000000000000 ) ) ;
#12420=DIRECTION ( 'NONE',  ( 0.000000000000000000, 0.000000000000000000, 1.000000000000000000 ) ) ;
#12428=CARTESIAN_POINT ( 'NONE',  ( -66.39923980726636898, 75.89776002577445979, -167.1454815528550739 ) ) ;
#12444=VERTEX_POINT ( 'NONE', #12455 ) ;
#12454=CARTESIAN_POINT ( 'NONE',  ( -57.08002265617300708, 84.22855780814606419, 15.00000000000006928 ) ) ;
#12455=CARTESIAN_POINT ( 'NONE',  ( -61.80899203128051056, 95.79950628479635100, -15.00000000000001421 ) ) ;
#12460=DIRECTION ( 'NONE',  ( 0.000000000000000000, 0.000000000000000000, 1.000000000000000000 ) ) ;
#12461=VERTEX_POINT ( 'NONE', #12650 ) ;
#12463=DIRECTION ( 'NONE',  ( -5.204170427930409450E-16, 0.000000000000000000, 1.000000000000000000 ) ) ;
#12464=EDGE_LOOP ( 'NONE', ( #14827, #1913, #8980, #17732 ) ) ;
#12467=ORIENTED_EDGE ( 'NONE', *, *, #2350, .F. ) ;
#12476=ORIENTED_EDGE ( 'NONE', *, *, #1820, .T. ) ;
#12482=EDGE_CURVE ( 'NONE', #12661, #1399, #7621, .T. ) ;
#12484=LINE ( 'NONE', #5263, #1209 ) ;
#12491=ORIENTED_EDGE ( 'NONE', *, *, #1148, .T. ) ;
#12501=DIRECTION ( 'NONE',  ( 1.156482317317869999E-16, 0.000000000000000000, 1.000000000000000000 ) ) ;
#12513=VERTEX_POINT ( 'NONE', #4118 ) ;
#12518=DIRECTION ( 'NONE',  ( 1.000000000000000000, 0.000000000000000000, 3.771137991253928573E-16 ) ) ;
#12520=DIRECTION ( 'NONE',  ( 1.156482317317869999E-16, 0.000000000000000000, 1.000000000000000000 ) ) ;
#12524=DIRECTION ( 'NONE',  ( -5.204170427930409450E-16, 0.000000000000000000, 1.000000000000000000 ) ) ;
#12525=CYLINDRICAL_SURFACE ( 'NONE', #14228, 10.24900000000001477 ) ;
#12536=CIRCLE ( 'NONE', #9525, 12.49999999999999112 ) ;
#12537=DIRECTION ( 'NONE',  ( 0.000000000000000000, 0.000000000000000000, 1.000000000000000000 ) ) ;
#12544=CYLINDRICAL_SURFACE ( 'NONE', #9716, 10.24900000000000055 ) ;
#12552=VECTOR ( 'NONE', #6552, 1000.000000000000000 ) ;
#12553=DIRECTION ( 'NONE',  ( 0.000000000000000000, 0.000000000000000000, 1.000000000000000000 ) ) ;
#12555=ORIENTED_EDGE ( 'NONE', *, *, #8477, .F. ) ;
#12567=CARTESIAN_POINT ( 'NONE',  ( -57.08002265617300708, 84.22855780814606419, -167.1454815528550739 ) ) ;
#12578=ORIENTED_EDGE ( 'NONE', *, *, #9755, .F. ) ;
#12580=MANIFOLD_SOLID_BREP ( 'Boss-Extrude15[2]', #17430 ) ;
#12598=ADVANCED_FACE ( 'NONE', ( #7292 ), #7732, .T. ) ;
#12600=DIRECTION ( 'NONE',  ( -5.204170427930409450E-16, 0.000000000000000000, 1.000000000000000000 ) ) ;
#12605=LINE ( 'NONE', #2486, #10585 ) ;
#12607=ADVANCED_FACE ( 'NONE', ( #12050 ), #11680, .T. ) ;
#12616=EDGE_CURVE ( 'NONE', #7041, #10126, #7635, .T. ) ;
#12617=DIRECTION ( 'NONE',  ( 0.000000000000000000, 0.000000000000000000, 1.000000000000000000 ) ) ;
#12622=ADVANCED_FACE ( 'NONE', ( #10646 ), #13356, .F. ) ;
#12624=CARTESIAN_POINT ( 'NONE',  ( -64.40194603863702127, 76.28065702765842104, -15.00000000000001421 ) ) ;
#12650=CARTESIAN_POINT ( 'NONE',  ( -63.34052343625892689, 73.40930968350525632, -15.00000000000001421 ) ) ;
#12651=CARTESIAN_POINT ( 'NONE',  ( -57.89103256796045116, 73.45256821284057480, -167.1454815528550739 ) ) ;
#12652=ORIENTED_EDGE ( 'NONE', *, *, #8115, .T. ) ;
#12657=LINE ( 'NONE', #11332, #11666 ) ;
#12658=AXIS2_PLACEMENT_3D ( 'NONE', #4142, #15549, #2646 ) ;
#12661=VERTEX_POINT ( 'NONE', #3248 ) ;
#12666=CARTESIAN_POINT ( 'NONE',  ( -51.34465738200551499, 92.72253132893560235, -15.00000000000001421 ) ) ;
#12673=VERTEX_POINT ( 'NONE', #11772 ) ;
#12679=EDGE_LOOP ( 'NONE', ( #15767, #8915, #7046, #6651 ) ) ;
#12689=ORIENTED_EDGE ( 'NONE', *, *, #13066, .T. ) ;
#12693=DIRECTION ( 'NONE',  ( -5.204170427930409450E-16, 0.000000000000000000, 1.000000000000000000 ) ) ;
#12696=VECTOR ( 'NONE', #7457, 1000.000000000000000 ) ;
#12697=ORIENTED_EDGE ( 'NONE', *, *, #3652, .F. ) ;
#12699=CARTESIAN_POINT ( 'NONE',  ( -57.08002265617300708, 84.22855780814606419, -15.00000000000001421 ) ) ;
#12716=LINE ( 'NONE', #18412, #4480 ) ;
#12719=DIRECTION ( 'NONE',  ( 1.000000000000000000, 0.000000000000000000, 5.551115123125777772E-16 ) ) ;
#12724=CARTESIAN_POINT ( 'NONE',  ( -46.69442755757756203, 81.24207102880484399, -15.00000000000001421 ) ) ;
#12726=ORIENTED_EDGE ( 'NONE', *, *, #5723, .T. ) ;
#12727=EDGE_CURVE ( 'NONE', #10691, #11670, #5831, .T. ) ;
#12728=EDGE_CURVE ( 'NONE', #4389, #2327, #16280, .T. ) ;
#12730=VECTOR ( 'NONE', #11033, 1000.000000000000000 ) ;
#12744=VECTOR ( 'NONE', #10018, 1000.000000000000000 ) ;
#12762=DIRECTION ( 'NONE',  ( 1.156482317317869999E-16, 0.000000000000000000, 1.000000000000000000 ) ) ;
#12766=ORIENTED_EDGE ( 'NONE', *, *, #5712, .F. ) ;
#12767=CARTESIAN_POINT ( 'NONE',  ( -47.27059076829218043, 81.25920652595885940, -15.00000000000001421 ) ) ;
#12772=DIRECTION ( 'NONE',  ( -5.204170427930409450E-16, 0.000000000000000000, 1.000000000000000000 ) ) ;
#12775=LINE ( 'NONE', #9673, #15383 ) ;
#12782=CARTESIAN_POINT ( 'NONE',  ( -61.80899203128051056, 95.79950628479635100, 15.00000000000006928 ) ) ;
#12783=VERTEX_POINT ( 'NONE', #8103 ) ;
#12789=ORIENTED_EDGE ( 'NONE', *, *, #6404, .T. ) ;
#12791=EDGE_CURVE ( 'NONE', #7041, #538, #821, .T. ) ;
#12793=ORIENTED_EDGE ( 'NONE', *, *, #5866, .T. ) ;
#12797=CARTESIAN_POINT ( 'NONE',  ( -47.59681378869034774, 80.34130291867735707, -167.1454815528550739 ) ) ;
#12798=CARTESIAN_POINT ( 'NONE',  ( -57.08002265617300708, 84.22855780814606419, -15.00000000000001421 ) ) ;
#12809=FACE_OUTER_BOUND ( 'NONE', #4102, .T. ) ;
#12810=EDGE_LOOP ( 'NONE', ( #6953, #17835, #9117, #4634 ) ) ;
#12813=ORIENTED_EDGE ( 'NONE', *, *, #12118, .T. ) ;
#12818=ADVANCED_FACE ( 'NONE', ( #2305 ), #12525, .T. ) ;
#12827=EDGE_CURVE ( 'NONE', #4520, #7041, #15991, .T. ) ;
#12838=EDGE_CURVE ( 'NONE', #4644, #15057, #16583, .T. ) ;
#12839=ADVANCED_FACE ( 'NONE', ( #2692 ), #14015, .T. ) ;
#12849=DIRECTION ( 'NONE',  ( 1.156482317317869999E-16, 0.000000000000000000, 1.000000000000000000 ) ) ;
#12851=CARTESIAN_POINT ( 'NONE',  ( -59.05157857372951469, 96.57209730311865314, 15.00000000000006928 ) ) ;
#12858=EDGE_CURVE ( 'NONE', #2137, #16012, #3539, .T. ) ;
#12861=CIRCLE ( 'NONE', #8669, 4.599999999999999645 ) ;
#12866=ORIENTED_EDGE ( 'NONE', *, *, #2650, .F. ) ;
#12870=DIRECTION ( 'NONE',  ( 1.000000000000000000, 0.000000000000000000, 0.000000000000000000 ) ) ;
#12886=ORIENTED_EDGE ( 'NONE', *, *, #3648, .T. ) ;
#12888=DIRECTION ( 'NONE',  ( 1.000000000000000000, 0.000000000000000000, 5.551115123125786646E-16 ) ) ;
#12889=CARTESIAN_POINT ( 'NONE',  ( -53.84898691462515785, 93.95493478196527803, -15.00000000000001421 ) ) ;
#12897=DIRECTION ( 'NONE',  ( 1.000000000000000000, 0.000000000000000000, 5.077734830647302671E-16 ) ) ;
#12899=EDGE_CURVE ( 'NONE', #4262, #9354, #11965, .T. ) ;
#12901=DIRECTION ( 'NONE',  ( -5.204170427930409450E-16, 0.000000000000000000, 1.000000000000000000 ) ) ;
#12903=DIRECTION ( 'NONE',  ( 1.000000000000000000, 0.000000000000000000, 0.000000000000000000 ) ) ;
#12904=CIRCLE ( 'NONE', #2424, 12.50000000000001776 ) ;
#12906=DIRECTION ( 'NONE',  ( 0.000000000000000000, 0.000000000000000000, 1.000000000000000000 ) ) ;
#12908=ORIENTED_EDGE ( 'NONE', *, *, #15098, .F. ) ;
#12920=( NAMED_UNIT ( * ) SI_UNIT ( $, .STERADIAN. ) SOLID_ANGLE_UNIT ( ) );
#12923=CARTESIAN_POINT ( 'NONE',  ( -52.04298920050707977, 93.78931001713317528, 15.00000000000006928 ) ) ;
#12926=CIRCLE ( 'NONE', #4820, 4.599999999999999645 ) ;
#12931=APPLICATION_CONTEXT ( 'automotive_design' ) ;
#12938=CARTESIAN_POINT ( 'NONE',  ( -48.74405704658271077, 91.10542963993684396, 15.00000000000006928 ) ) ;
#12948=CIRCLE ( 'NONE', #11150, 4.599999999999992539 ) ;
#12951=EDGE_CURVE ( 'NONE', #13256, #12444, #13038, .T. ) ;
#12956=ORIENTED_EDGE ( 'NONE', *, *, #8594, .F. ) ;
#12970=DIRECTION ( 'NONE',  ( 0.000000000000000000, 0.000000000000000000, 1.000000000000000000 ) ) ;
#12975=ORIENTED_EDGE ( 'NONE', *, *, #11897, .F. ) ;
#12977=VECTOR ( 'NONE', #2322, 1000.000000000000000 ) ;
#12978=VECTOR ( 'NONE', #11936, 1000.000000000000000 ) ;
#12984=VECTOR ( 'NONE', #9056, 1000.000000000000000 ) ;
#12996=DIRECTION ( 'NONE',  ( 1.000000000000000000, 0.000000000000000000, 3.771137991253923150E-16 ) ) ;
#13002=AXIS2_PLACEMENT_3D ( 'NONE', #3739, #15137, #7575 ) ;
#13012=CARTESIAN_POINT ( 'NONE',  ( -57.08002265617300708, 84.22855780814606419, 15.00000000000006928 ) ) ;
#13017=CARTESIAN_POINT ( 'NONE',  ( -57.08002265617300708, 84.22855780814606419, -15.00000000000001421 ) ) ;
#13020=CARTESIAN_POINT ( 'NONE',  ( -53.53072411395612562, 94.43552448259771381, 15.00000000000006928 ) ) ;
#13035=CARTESIAN_POINT ( 'NONE',  ( -57.08002265617300708, 84.22855780814606419, -15.00000000000001421 ) ) ;
#13038=CIRCLE ( 'NONE', #10290, 4.600000000000006750 ) ;
#13059=CARTESIAN_POINT ( 'NONE',  ( -61.98305514952129158, 93.22868410554717400, -15.00000000000001421 ) ) ;
#13061=CARTESIAN_POINT ( 'NONE',  ( -57.99147934508202695, 74.02016676429184372, 15.00000000000006928 ) ) ;
#13066=EDGE_CURVE ( 'NONE', #15720, #2855, #17078, .T. ) ;
#13076=CARTESIAN_POINT ( 'NONE',  ( -61.98611128973170992, 74.59995546124152099, 15.00000000000006928 ) ) ;
#13085=EDGE_CURVE ( 'NONE', #9307, #4088, #12605, .T. ) ;
#13098=CARTESIAN_POINT ( 'NONE',  ( -66.88945454405379110, 81.25920652595873150, 15.00000000000006928 ) ) ;
#13100=DIRECTION ( 'NONE',  ( 1.000000000000000000, 0.000000000000000000, 3.771137991253934490E-16 ) ) ;
#13103=ORIENTED_EDGE ( 'NONE', *, *, #8486, .T. ) ;
#13106=DIRECTION ( 'NONE',  ( 1.156482317317869999E-16, 0.000000000000000000, 1.000000000000000000 ) ) ;
#13119=DIRECTION ( 'NONE',  ( 1.156482317317869999E-16, 0.000000000000000000, 1.000000000000000000 ) ) ;
#13121=ORIENTED_EDGE ( 'NONE', *, *, #6169, .F. ) ;
#13128=EDGE_LOOP ( 'NONE', ( #8514, #11514, #458, #13551 ) ) ;
#13132=CARTESIAN_POINT ( 'NONE',  ( -52.17393402261416213, 74.59995546124159205, -15.00000000000001421 ) ) ;
#13139=VECTOR ( 'NONE', #3046, 1000.000000000000000 ) ;
#13147=CARTESIAN_POINT ( 'NONE',  ( -57.74389692835771370, 95.01461175692088545, -167.1454815528550739 ) ) ;
#13158=LINE ( 'NONE', #15783, #10600 ) ;
#13166=ORIENTED_EDGE ( 'NONE', *, *, #3652, .T. ) ;
#13171=DIRECTION ( 'NONE',  ( 0.000000000000000000, 0.000000000000000000, 1.000000000000000000 ) ) ;
#13181=DIRECTION ( 'NONE',  ( 0.000000000000000000, 0.000000000000000000, 1.000000000000000000 ) ) ;
#13182=DIRECTION ( 'NONE',  ( 0.000000000000000000, 0.000000000000000000, 1.000000000000000000 ) ) ;
#13186=CARTESIAN_POINT ( 'NONE',  ( -69.56651066787533466, 84.80960611389535586, -167.1454815528550739 ) ) ;
#13190=VERTEX_POINT ( 'NONE', #8111 ) ;
#13193=ORIENTED_EDGE ( 'NONE', *, *, #2311, .T. ) ;
#13196=DIRECTION ( 'NONE',  ( -5.204170427930409450E-16, 0.000000000000000000, 1.000000000000000000 ) ) ;
#13203=ORIENTED_EDGE ( 'NONE', *, *, #6885, .F. ) ;
#13204=FACE_OUTER_BOUND ( 'NONE', #11280, .T. ) ;
#13209=AXIS2_PLACEMENT_3D ( 'NONE', #5936, #15959, #3153 ) ;
#13213=ORIENTED_EDGE ( 'NONE', *, *, #12827, .F. ) ;
#13216=AXIS2_PLACEMENT_3D ( 'NONE', #1825, #5084, #15003 ) ;
#13217=CYLINDRICAL_SURFACE ( 'NONE', #7600, 10.24900000000000055 ) ;
#13222=AXIS2_PLACEMENT_3D ( 'NONE', #9189, #6457, #14879 ) ;
#13226=DIRECTION ( 'NONE',  ( 0.000000000000000000, 0.000000000000000000, 1.000000000000000000 ) ) ;
#13228=CARTESIAN_POINT ( 'NONE',  ( -44.89980253466632831, 81.41924511788819530, -15.00000000000001421 ) ) ;
#13231=ORIENTED_EDGE ( 'NONE', *, *, #2255, .T. ) ;
#13241=DIRECTION ( 'NONE',  ( 0.000000000000000000, 0.000000000000000000, 1.000000000000000000 ) ) ;
#13252=CARTESIAN_POINT ( 'NONE',  ( -57.08002265617300708, 84.22855780814606419, -167.1454815528550739 ) ) ;
#13256=VERTEX_POINT ( 'NONE', #17650 ) ;
#13262=DIRECTION ( 'NONE',  ( 0.000000000000000000, 0.000000000000000000, 1.000000000000000000 ) ) ;
#13265=FACE_OUTER_BOUND ( 'NONE', #15534, .T. ) ;
#13272=FACE_OUTER_BOUND ( 'NONE', #8279, .T. ) ;
#13274=AXIS2_PLACEMENT_3D ( 'NONE', #11212, #2960, #14011 ) ;
#13278=EDGE_CURVE ( 'NONE', #9072, #16289, #16337, .T. ) ;
#13282=EDGE_CURVE ( 'NONE', #11356, #14710, #5217, .T. ) ;
#13289=AXIS2_PLACEMENT_3D ( 'NONE', #6112, #11839, #4628 ) ;
#13291=CARTESIAN_POINT ( 'NONE',  ( -44.59353464447068660, 84.80960611389554060, -15.00000000000001421 ) ) ;
#13293=CYLINDRICAL_SURFACE ( 'NONE', #17584, 4.600000000000006750 ) ;
#13300=CARTESIAN_POINT ( 'NONE',  ( -44.63071506687145984, 85.35316464920607871, -15.00000000000001421 ) ) ;
#13309=ORIENTED_EDGE ( 'NONE', *, *, #14873, .T. ) ;
#13310=ADVANCED_FACE ( 'NONE', ( #13646 ), #6515, .T. ) ;
#13312=FACE_OUTER_BOUND ( 'NONE', #6823, .T. ) ;
#13313=DIRECTION ( 'NONE',  ( 0.000000000000000000, 0.000000000000000000, 1.000000000000000000 ) ) ;
#13323=ORIENTED_EDGE ( 'NONE', *, *, #18306, .F. ) ;
#13325=ORIENTED_EDGE ( 'NONE', *, *, #14201, .F. ) ;
#13326=CARTESIAN_POINT ( 'NONE',  ( -65.41598826576338865, 91.10542963993673027, -167.1454815528550739 ) ) ;
#13333=DIRECTION ( 'NONE',  ( 1.000000000000000000, 0.000000000000000000, 3.771137991253923150E-16 ) ) ;
#13339=DIRECTION ( 'NONE',  ( 0.000000000000000000, 0.000000000000000000, 1.000000000000000000 ) ) ;
#13342=CARTESIAN_POINT ( 'NONE',  ( -46.65463807863145007, 87.07303407725225952, -15.00000000000001421 ) ) ;
#13346=ORIENTED_EDGE ( 'NONE', *, *, #6889, .T. ) ;
#13351=DIRECTION ( 'NONE',  ( 1.000000000000000000, 0.000000000000000000, 4.625929269271485914E-16 ) ) ;
#13356=CYLINDRICAL_SURFACE ( 'NONE', #8837, 7.500000000000000000 ) ;
#13365=ORIENTED_EDGE ( 'NONE', *, *, #4452, .T. ) ;
#13375=DIRECTION ( 'NONE',  ( 1.000000000000000000, 0.000000000000000000, 0.000000000000000000 ) ) ;
#13379=DIRECTION ( 'NONE',  ( 1.000000000000000000, 0.000000000000000000, 0.000000000000000000 ) ) ;
#13384=CARTESIAN_POINT ( 'NONE',  ( -44.63071506687145984, 85.35316464920607871, -167.1454815528550739 ) ) ;
#13385=ORIENTED_EDGE ( 'NONE', *, *, #17708, .T. ) ;
#13399=AXIS2_PLACEMENT_3D ( 'NONE', #1419, #7301, #4481 ) ;
#13402=CARTESIAN_POINT ( 'NONE',  ( -50.35400969968294049, 73.69239390902568232, -15.00000000000001421 ) ) ;
#13408=ORIENTED_EDGE ( 'NONE', *, *, #14155, .F. ) ;
#13422=CIRCLE ( 'NONE', #4753, 4.600000000000006750 ) ;
#13429=ORIENTED_EDGE ( 'NONE', *, *, #10398, .F. ) ;
#13430=ORIENTED_EDGE ( 'NONE', *, *, #10856, .T. ) ;
#13432=CYLINDRICAL_SURFACE ( 'NONE', #4585, 12.49999999999999112 ) ;
#13433=ADVANCED_FACE ( 'NONE', ( #8217 ), #8306, .T. ) ;
#13434=LINE ( 'NONE', #6415, #13835 ) ;
#13435=ORIENTED_EDGE ( 'NONE', *, *, #489, .F. ) ;
#13437=SHAPE_DEFINITION_REPRESENTATION ( #10890, #15047 ) ;
#13438=FACE_OUTER_BOUND ( 'NONE', #2596, .T. ) ;
#13439=( NAMED_UNIT ( * ) PLANE_ANGLE_UNIT ( ) SI_UNIT ( $, .RADIAN. ) );
#13441=CARTESIAN_POINT ( 'NONE',  ( -56.80760832784252301, 71.73152654333280509, -167.1454815528550739 ) ) ;
#13444=DIRECTION ( 'NONE',  ( 1.000000000000000000, 0.000000000000000000, 0.000000000000000000 ) ) ;
#13446=CARTESIAN_POINT ( 'NONE',  ( -57.08002265617300708, 84.22855780814606419, -167.1454815528550739 ) ) ;
#13451=DIRECTION ( 'NONE',  ( -5.204170427930409450E-16, 0.000000000000000000, 1.000000000000000000 ) ) ;
#13453=ORIENTED_EDGE ( 'NONE', *, *, #1042, .T. ) ;
#13454=CARTESIAN_POINT ( 'NONE',  ( -57.08002265617300708, 84.22855780814606419, -167.1454815528550739 ) ) ;
#13461=CIRCLE ( 'NONE', #4205, 4.599999999999992539 ) ;
#13473=DIRECTION ( 'NONE',  ( -5.204170427930409450E-16, 0.000000000000000000, 1.000000000000000000 ) ) ;
#13474=EDGE_CURVE ( 'NONE', #16963, #9640, #447, .T. ) ;
#13476=DIRECTION ( 'NONE',  ( 0.000000000000000000, 0.000000000000000000, 1.000000000000000000 ) ) ;
#13477=ORIENTED_EDGE ( 'NONE', *, *, #6404, .F. ) ;
#13478=CYLINDRICAL_SURFACE ( 'NONE', #6727, 10.24900000000000055 ) ;
#13481=CIRCLE ( 'NONE', #6291, 10.24899999999999345 ) ;
#13483=EDGE_CURVE ( 'NONE', #4200, #7349, #13158, .T. ) ;
#13485=EDGE_CURVE ( 'NONE', #12673, #4970, #8214, .T. ) ;
#13486=CARTESIAN_POINT ( 'NONE',  ( -57.08002265617300708, 84.22855780814606419, -15.00000000000001421 ) ) ;
#13488=CARTESIAN_POINT ( 'NONE',  ( -57.08002265617300708, 84.22855780814606419, -167.1454815528550739 ) ) ;
#13498=DIRECTION ( 'NONE',  ( 0.000000000000000000, 0.000000000000000000, 1.000000000000000000 ) ) ;
#13507=ADVANCED_FACE ( 'NONE', ( #7538 ), #249, .T. ) ;
#13509=ADVANCED_FACE ( 'NONE', ( #6120 ), #4715, .T. ) ;
#13510=ORIENTED_EDGE ( 'NONE', *, *, #17104, .F. ) ;
#13513=EDGE_CURVE ( 'NONE', #2837, #18489, #4044, .T. ) ;
#13516=ORIENTED_EDGE ( 'NONE', *, *, #3442, .F. ) ;
#13519=VERTEX_POINT ( 'NONE', #8592 ) ;
#13530=ORIENTED_EDGE ( 'NONE', *, *, #11735, .F. ) ;
#13531=VECTOR ( 'NONE', #526, 1000.000000000000000 ) ;
#13534=DIRECTION ( 'NONE',  ( 1.000000000000000000, 0.000000000000000000, 3.771137991253934490E-16 ) ) ;
#13538=CYLINDRICAL_SURFACE ( 'NONE', #16282, 4.599999999999999645 ) ;
#13541=CARTESIAN_POINT ( 'NONE',  ( -58.51182448057780050, 96.64628479562776420, -167.1454815528550739 ) ) ;
#13546=DIRECTION ( 'NONE',  ( 1.000000000000000000, 0.000000000000000000, 0.000000000000000000 ) ) ;
#13551=ORIENTED_EDGE ( 'NONE', *, *, #16444, .F. ) ;
#13552=DIRECTION ( 'NONE',  ( 0.000000000000000000, 0.000000000000000000, 1.000000000000000000 ) ) ;
#13557=ORIENTED_EDGE ( 'NONE', *, *, #4121, .T. ) ;
#13565=FACE_OUTER_BOUND ( 'NONE', #15880, .T. ) ;
#13572=ADVANCED_FACE ( 'NONE', ( #4639 ), #11658, .T. ) ;
#13575=DIRECTION ( 'NONE',  ( -1.000000000000000000, -4.062187864517847658E-15, 1.692578276882436442E-16 ) ) ;
#13587=AXIS2_PLACEMENT_3D ( 'NONE', #8640, #1532, #7239 ) ;
#13591=ORIENTED_EDGE ( 'NONE', *, *, #3446, .F. ) ;
#13593=CARTESIAN_POINT ( 'NONE',  ( -63.16290507965269541, 75.97988867778799715, -167.1454815528550739 ) ) ;
#13610=LINE ( 'NONE', #10616, #10831 ) ;
#13616=EDGE_CURVE ( 'NONE', #2018, #2837, #17465, .T. ) ;
#13621=ORIENTED_EDGE ( 'NONE', *, *, #12482, .T. ) ;
#13643=DIRECTION ( 'NONE',  ( 0.000000000000000000, 0.000000000000000000, 1.000000000000000000 ) ) ;
#13646=FACE_OUTER_BOUND ( 'NONE', #6545, .T. ) ;
#13662=FACE_OUTER_BOUND ( 'NONE', #8113, .T. ) ;
#13663=EDGE_LOOP ( 'NONE', ( #18248, #12052, #12491, #7984 ) ) ;
#13667=ORIENTED_EDGE ( 'NONE', *, *, #2650, .T. ) ;
#13671=ORIENTED_EDGE ( 'NONE', *, *, #6814, .T. ) ;
#13673=CARTESIAN_POINT ( 'NONE',  ( -51.85133027979232878, 95.58244595420329404, 15.00000000000006928 ) ) ;
#13674=DIRECTION ( 'NONE',  ( -1.000000000000000000, 0.000000000000000000, 1.387778780781445182E-16 ) ) ;
#13675=EDGE_CURVE ( 'NONE', #11552, #15366, #9105, .T. ) ;
#13677=CARTESIAN_POINT ( 'NONE',  ( -57.08002265617300708, 84.22855780814606419, -15.00000000000001421 ) ) ;
#13694=EDGE_LOOP ( 'NONE', ( #3836, #14854, #2333, #7634 ) ) ;
#13705=EDGE_CURVE ( 'NONE', #3974, #13190, #4911, .T. ) ;
#13712=LINE ( 'NONE', #2296, #10540 ) ;
#13715=DIRECTION ( 'NONE',  ( 0.000000000000000000, 0.000000000000000000, 1.000000000000000000 ) ) ;
#13719=ORIENTED_EDGE ( 'NONE', *, *, #17610, .T. ) ;
#13723=DIRECTION ( 'NONE',  ( 1.000000000000000000, 0.000000000000000000, 5.077734830647302671E-16 ) ) ;
#13747=DIRECTION ( 'NONE',  ( 0.000000000000000000, 0.000000000000000000, 1.000000000000000000 ) ) ;
#13748=CARTESIAN_POINT ( 'NONE',  ( -62.11705611183893438, 93.78931001713317528, 15.00000000000006928 ) ) ;
#13749=CARTESIAN_POINT ( 'NONE',  ( -57.08002265617300708, 84.22855780814606419, -15.00000000000001421 ) ) ;
#13750=VERTEX_POINT ( 'NONE', #14092 ) ;
#13766=VECTOR ( 'NONE', #12617, 1000.000000000000000 ) ;
#13769=DIRECTION ( 'NONE',  ( 1.000000000000000000, 0.000000000000000000, 5.077734830647306615E-16 ) ) ;
#13783=AXIS2_PLACEMENT_3D ( 'NONE', #15180, #3582, #979 ) ;
#13786=PRODUCT_DEFINITION ( 'UNKNOWN', '', #7580, #10962 ) ;
#13788=AXIS2_PLACEMENT_3D ( 'NONE', #11902, #5997, #6091 ) ;
#13790=VERTEX_POINT ( 'NONE', #5899 ) ;
#13801=CARTESIAN_POINT ( 'NONE',  ( -48.99724571598702738, 77.92691374209489652, -167.1454815528550739 ) ) ;
#13810=DIRECTION ( 'NONE',  ( -1.000000000000000000, 0.000000000000000000, 0.000000000000000000 ) ) ;
#13811=AXIS2_PLACEMENT_3D ( 'NONE', #15385, #11180, #8176 ) ;
#13812=ORIENTED_EDGE ( 'NONE', *, *, #8914, .F. ) ;
#13813=EDGE_CURVE ( 'NONE', #1187, #6109, #16784, .T. ) ;
#13819=FACE_OUTER_BOUND ( 'NONE', #5586, .T. ) ;
#13821=CIRCLE ( 'NONE', #7255, 4.599999999999992539 ) ;
#13822=DIRECTION ( 'NONE',  ( 0.000000000000000000, 0.000000000000000000, 1.000000000000000000 ) ) ;
#13824=DIRECTION ( 'NONE',  ( -5.204170427930409450E-16, 0.000000000000000000, 1.000000000000000000 ) ) ;
#13835=VECTOR ( 'NONE', #10537, 1000.000000000000000 ) ;
#13840=EDGE_CURVE ( 'NONE', #8753, #12673, #15708, .T. ) ;
#13843=CARTESIAN_POINT ( 'NONE',  ( -65.94558993203320085, 89.37090336996871542, 15.00000000000006928 ) ) ;
#13844=AXIS2_PLACEMENT_3D ( 'NONE', #15414, #12520, #4094 ) ;
#13853=CARTESIAN_POINT ( 'NONE',  ( -62.30871503255384170, 95.58244595420320877, 15.00000000000006928 ) ) ;
#13861=ORIENTED_EDGE ( 'NONE', *, *, #16791, .F. ) ;
#13865=AXIS2_PLACEMENT_3D ( 'NONE', #3716, #16327, #6504 ) ;
#13884=AXIS2_PLACEMENT_3D ( 'NONE', #14816, #3149, #2190 ) ;
#13886=ORIENTED_EDGE ( 'NONE', *, *, #17502, .T. ) ;
#13890=DIRECTION ( 'NONE',  ( 1.156482317317869999E-16, 0.000000000000000000, 1.000000000000000000 ) ) ;
#13894=VERTEX_POINT ( 'NONE', #16009 ) ;
#13897=CIRCLE ( 'NONE', #3416, 12.50000000000000355 ) ;
#13913=ORIENTED_EDGE ( 'NONE', *, *, #1563, .T. ) ;
#13914=CARTESIAN_POINT ( 'NONE',  ( -60.71187100093244737, 74.64462966772953223, -167.1454815528550739 ) ) ;
#13915=CARTESIAN_POINT ( 'NONE',  ( -59.37303238940180705, 94.21775734381046163, -15.00000000000001421 ) ) ;
#13925=DIRECTION ( 'NONE',  ( -1.000000000000000000, 0.000000000000000000, 0.000000000000000000 ) ) ;
#13931=DIRECTION ( 'NONE',  ( 1.000000000000000000, 0.000000000000000000, 0.000000000000000000 ) ) ;
#13937=DIRECTION ( 'NONE',  ( -1.000000000000000000, 3.016910393003147592E-15, 0.000000000000000000 ) ) ;
#13938=CYLINDRICAL_SURFACE ( 'NONE', #9418, 4.599999999999999645 ) ;
#13945=CARTESIAN_POINT ( 'NONE',  ( -61.98305514952129158, 93.22868410554717400, 15.00000000000006928 ) ) ;
#13946=ORIENTED_EDGE ( 'NONE', *, *, #13840, .T. ) ;
#13947=CARTESIAN_POINT ( 'NONE',  ( -52.04298920050707977, 93.78931001713317528, -15.00000000000001421 ) ) ;
#13952=CYLINDRICAL_SURFACE ( 'NONE', #1164, 10.24900000000000055 ) ;
#13955=EDGE_LOOP ( 'NONE', ( #5646, #4865, #16091, #9917 ) ) ;
#13964=ADVANCED_FACE ( 'NONE', ( #10479 ), #13478, .T. ) ;
#13969=FACE_OUTER_BOUND ( 'NONE', #16933, .T. ) ;
#13971=ORIENTED_EDGE ( 'NONE', *, *, #14155, .T. ) ;
#13972=CARTESIAN_POINT ( 'NONE',  ( -63.34052343625892689, 73.40930968350525632, 15.00000000000006928 ) ) ;
#13977=EDGE_CURVE ( 'NONE', #1187, #14698, #2560, .T. ) ;
#13989=EDGE_CURVE ( 'NONE', #10224, #12513, #9119, .T. ) ;
#13994=CARTESIAN_POINT ( 'NONE',  ( -46.27380910617147691, 84.15481808402802244, 15.00000000000009592 ) ) ;
#13997=ORIENTED_EDGE ( 'NONE', *, *, #7443, .F. ) ;
#14001=DIRECTION ( 'NONE',  ( -5.204170427930409450E-16, 0.000000000000000000, 1.000000000000000000 ) ) ;
#14005=ORIENTED_EDGE ( 'NONE', *, *, #7113, .F. ) ;
#14007=ORIENTED_EDGE ( 'NONE', *, *, #13483, .T. ) ;
#14011=DIRECTION ( 'NONE',  ( -1.000000000000000000, 0.000000000000000000, 0.000000000000000000 ) ) ;
#14014=CYLINDRICAL_SURFACE ( 'NONE', #3452, 4.599999999999999645 ) ;
#14015=CYLINDRICAL_SURFACE ( 'NONE', #14753, 10.24900000000000766 ) ;
#14023=CARTESIAN_POINT ( 'NONE',  ( -54.75080917176597950, 94.79374675277695417, -167.1454815528550739 ) ) ;
#14033=CARTESIAN_POINT ( 'NONE',  ( -50.99714023269321217, 75.97988867778809663, 15.00000000000006928 ) ) ;
#14034=DIRECTION ( 'NONE',  ( -5.204170427930409450E-16, 0.000000000000000000, 1.000000000000000000 ) ) ;
#14039=ORIENTED_EDGE ( 'NONE', *, *, #7355, .F. ) ;
#14044=CIRCLE ( 'NONE', #4461, 4.599999999999992539 ) ;
#14047=ORIENTED_EDGE ( 'NONE', *, *, #16248, .F. ) ;
#14055=DIRECTION ( 'NONE',  ( 0.000000000000000000, 0.000000000000000000, 1.000000000000000000 ) ) ;
#14060=ORIENTED_EDGE ( 'NONE', *, *, #5956, .T. ) ;
#14083=ORIENTED_EDGE ( 'NONE', *, *, #11473, .T. ) ;
#14084=CARTESIAN_POINT ( 'NONE',  ( -57.08002265617300708, 84.22855780814606419, -167.1454815528550739 ) ) ;
#14092=CARTESIAN_POINT ( 'NONE',  ( -60.18936887439735273, 72.12145385653096241, -15.00000000000001421 ) ) ;
#14097=ADVANCED_FACE ( 'NONE', ( #2629 ), #14140, .T. ) ;
#14099=AXIS2_PLACEMENT_3D ( 'NONE', #10345, #17258, #7627 ) ;
#14104=ORIENTED_EDGE ( 'NONE', *, *, #12482, .F. ) ;
#14106=DIRECTION ( 'NONE',  ( -1.000000000000000000, 5.416250486023796615E-15, 1.692578276882436442E-16 ) ) ;
#14107=DIRECTION ( 'NONE',  ( 0.000000000000000000, 0.000000000000000000, 1.000000000000000000 ) ) ;
#14108=CARTESIAN_POINT ( 'NONE',  ( -49.58002265617300708, 84.22855780814606419, 15.00000000000007283 ) ) ;
#14111=DIRECTION ( 'NONE',  ( -1.000000000000000000, 3.016910393003138520E-15, 0.000000000000000000 ) ) ;
#14124=AXIS2_PLACEMENT_3D ( 'NONE', #16909, #15215, #11021 ) ;
#14128=LINE ( 'NONE', #15517, #12730 ) ;
#14133=CARTESIAN_POINT ( 'NONE',  ( -57.08002265617300708, 84.22855780814606419, 15.00000000000006928 ) ) ;
#14136=AXIS2_PLACEMENT_3D ( 'NONE', #17890, #5073, #3686 ) ;
#14137=CARTESIAN_POINT ( 'NONE',  ( -69.37109144396066540, 81.95267818613797317, -167.1454815528550739 ) ) ;
#14139=CIRCLE ( 'NONE', #11736, 12.50000000000000355 ) ;
#14140=CYLINDRICAL_SURFACE ( 'NONE', #4765, 4.599999999999999645 ) ;
#14141=AXIS2_PLACEMENT_3D ( 'NONE', #11905, #7509, #5837 ) ;
#14151=DIRECTION ( 'NONE',  ( 0.000000000000000000, 0.000000000000000000, 1.000000000000000000 ) ) ;
#14155=EDGE_CURVE ( 'NONE', #15720, #18116, #13, .T. ) ;
#14157=ORIENTED_EDGE ( 'NONE', *, *, #7306, .T. ) ;
#14159=DIRECTION ( 'NONE',  ( -1.000000000000000000, 0.000000000000000000, 0.000000000000000000 ) ) ;
#14160=VERTEX_POINT ( 'NONE', #9745 ) ;
#14161=AXIS2_PLACEMENT_3D ( 'NONE', #10678, #9460, #15154 ) ;
#14162=LINE ( 'NONE', #1698, #16659 ) ;
#14168=VERTEX_POINT ( 'NONE', #18249 ) ;
#14183=AXIS2_PLACEMENT_3D ( 'NONE', #14570, #17463, #12046 ) ;
#14185=VECTOR ( 'NONE', #13313, 1000.000000000000000 ) ;
#14193=VECTOR ( 'NONE', #16255, 1000.000000000000000 ) ;
#14201=EDGE_CURVE ( 'NONE', #18427, #12358, #12657, .T. ) ;
#14215=AXIS2_PLACEMENT_3D ( 'NONE', #14133, #7379, #5691 ) ;
#14228=AXIS2_PLACEMENT_3D ( 'NONE', #2218, #5013, #10726 ) ;
#14231=CARTESIAN_POINT ( 'NONE',  ( -127.5926225674732279, 47.87487112387803023, 15.00000000000004263 ) ) ;
#14237=CYLINDRICAL_SURFACE ( 'NONE', #968, 10.24899999999999345 ) ;
#14238=ORIENTED_EDGE ( 'NONE', *, *, #1933, .T. ) ;
#14241=ORIENTED_EDGE ( 'NONE', *, *, #12838, .F. ) ;
#14250=CARTESIAN_POINT ( 'NONE',  ( -45.85876501399108207, 78.72098330317804482, -15.00000000000001421 ) ) ;
#14259=FACE_OUTER_BOUND ( 'NONE', #805, .T. ) ;
#14268=ORIENTED_EDGE ( 'NONE', *, *, #11765, .F. ) ;
#14271=ORIENTED_EDGE ( 'NONE', *, *, #18277, .T. ) ;
#14272=DIRECTION ( 'NONE',  ( 1.000000000000000000, 0.000000000000000000, 3.771137991253928573E-16 ) ) ;
#14273=FACE_OUTER_BOUND ( 'NONE', #16299, .T. ) ;
#14286=DIRECTION ( 'NONE',  ( 1.000000000000000000, 0.000000000000000000, 0.000000000000000000 ) ) ;
#14291=EDGE_CURVE ( 'NONE', #8437, #2855, #5083, .T. ) ;
#14297=CIRCLE ( 'NONE', #6509, 12.50000000000000355 ) ;
#14300=ORIENTED_EDGE ( 'NONE', *, *, #5866, .F. ) ;
#14303=EDGE_CURVE ( 'NONE', #768, #3406, #6259, .T. ) ;
#14305=CYLINDRICAL_SURFACE ( 'NONE', #6730, 4.599999999999992539 ) ;
#14310=ADVANCED_FACE ( 'NONE', ( #17557 ), #195, .T. ) ;
#14311=DIRECTION ( 'NONE',  ( -5.204170427930409450E-16, 0.000000000000000000, 1.000000000000000000 ) ) ;
#14316=VERTEX_POINT ( 'NONE', #5882 ) ;
#14319=VERTEX_POINT ( 'NONE', #11601 ) ;
#14333=DIRECTION ( 'NONE',  ( 0.000000000000000000, 0.000000000000000000, 1.000000000000000000 ) ) ;
#14335=FACE_OUTER_BOUND ( 'NONE', #3754, .T. ) ;
#14345=CIRCLE ( 'NONE', #2091, 12.49999999999999112 ) ;
#14354=CIRCLE ( 'NONE', #15239, 10.24900000000000055 ) ;
#14362=ORIENTED_EDGE ( 'NONE', *, *, #972, .F. ) ;
#14366=VERTEX_POINT ( 'NONE', #5116 ) ;
#14369=CARTESIAN_POINT ( 'NONE',  ( -50.24148097183213935, 76.59466308582166505, 15.00000000000009592 ) ) ;
#14372=DIRECTION ( 'NONE',  ( 1.156482317317869999E-16, 0.000000000000000000, 1.000000000000000000 ) ) ;
#14374=LINE ( 'NONE', #8862, #2409 ) ;
#14375=FACE_OUTER_BOUND ( 'NONE', #9834, .T. ) ;
#14379=CARTESIAN_POINT ( 'NONE',  ( -60.76828531927866095, 74.07097899412299569, 15.00000000000006928 ) ) ;
#14396=AXIS2_PLACEMENT_3D ( 'NONE', #17922, #13824, #13723 ) ;
#14407=AXIS2_PLACEMENT_3D ( 'NONE', #12724, #4000, #8402 ) ;
#14410=ORIENTED_EDGE ( 'NONE', *, *, #9637, .T. ) ;
#14427=ADVANCED_FACE ( 'NONE', ( #14848 ), #7740, .F. ) ;
#14428=CARTESIAN_POINT ( 'NONE',  ( -67.88623620617454435, 84.15481808402788033, 15.00000000000006928 ) ) ;
#14429=ORIENTED_EDGE ( 'NONE', *, *, #16581, .F. ) ;
#14433=EDGE_CURVE ( 'NONE', #16418, #2884, #6329, .T. ) ;
#14436=DIRECTION ( 'NONE',  ( -5.204170427930409450E-16, 0.000000000000000000, 1.000000000000000000 ) ) ;
#14442=CIRCLE ( 'NONE', #3362, 12.50000000000000355 ) ;
#14452=DIRECTION ( 'NONE',  ( -1.000000000000000000, -3.016910393003147592E-15, 0.000000000000000000 ) ) ;
#14455=DIRECTION ( 'NONE',  ( 0.000000000000000000, 0.000000000000000000, 1.000000000000000000 ) ) ;
#14462=CARTESIAN_POINT ( 'NONE',  ( -57.08002265617300708, 84.22855780814606419, -167.1454815528550739 ) ) ;
#14468=CARTESIAN_POINT ( 'NONE',  ( -54.95363092160842911, 73.63336328296981037, -167.1454815528550739 ) ) ;
#14471=CYLINDRICAL_SURFACE ( 'NONE', #6920, 4.599999999999992539 ) ;
#14483=CYLINDRICAL_SURFACE ( 'NONE', #3364, 4.599999999999992539 ) ;
#14485=CIRCLE ( 'NONE', #7910, 10.24900000000000766 ) ;
#14490=AXIS2_PLACEMENT_3D ( 'NONE', #12231, #16525, #13931 ) ;
#14495=CIRCLE ( 'NONE', #14215, 12.50000000000000355 ) ;
#14498=DIRECTION ( 'NONE',  ( -5.204170427930409450E-16, 0.000000000000000000, 1.000000000000000000 ) ) ;
#14503=ORIENTED_EDGE ( 'NONE', *, *, #17842, .F. ) ;
#14506=CIRCLE ( 'NONE', #5243, 4.600000000000006750 ) ;
#14520=ORIENTED_EDGE ( 'NONE', *, *, #828, .F. ) ;
#14523=ADVANCED_FACE ( 'NONE', ( #1117 ), #4007, .T. ) ;
#14528=DIRECTION ( 'NONE',  ( 1.156482317317869999E-16, 0.000000000000000000, 1.000000000000000000 ) ) ;
#14536=ADVANCED_FACE ( 'NONE', ( #15714 ), #11128, .T. ) ;
#14537=CARTESIAN_POINT ( 'NONE',  ( -66.02736529514692165, 75.49957964911740760, 15.00000000000006928 ) ) ;
#14538=EDGE_CURVE ( 'NONE', #616, #18359, #9583, .T. ) ;
#14541=ORIENTED_EDGE ( 'NONE', *, *, #16691, .T. ) ;
#14545=ORIENTED_EDGE ( 'NONE', *, *, #14303, .T. ) ;
#14553=DIRECTION ( 'NONE',  ( 1.000000000000000000, 0.000000000000000000, 0.000000000000000000 ) ) ;
#14558=DIRECTION ( 'NONE',  ( 1.156482317317869999E-16, 0.000000000000000000, 1.000000000000000000 ) ) ;
#14559=ORIENTED_EDGE ( 'NONE', *, *, #18438, .F. ) ;
#14560=DIRECTION ( 'NONE',  ( 0.000000000000000000, 0.000000000000000000, 1.000000000000000000 ) ) ;
#14565=DIRECTION ( 'NONE',  ( 1.000000000000000000, 0.000000000000000000, 0.000000000000000000 ) ) ;
#14569=CARTESIAN_POINT ( 'NONE',  ( -49.93060289285580922, 91.57211267264388255, 15.00000000000006928 ) ) ;
#14570=CARTESIAN_POINT ( 'NONE',  ( -65.41598826576338865, 91.10542963993673027, 15.00000000000006928 ) ) ;
#14575=DIRECTION ( 'NONE',  ( 1.000000000000000000, 0.000000000000000000, 0.000000000000000000 ) ) ;
#14589=CARTESIAN_POINT ( 'NONE',  ( -47.88529808651028929, 78.55081803573747834, -167.1454815528550739 ) ) ;
#14609=ORIENTED_EDGE ( 'NONE', *, *, #18201, .T. ) ;
#14610=ORIENTED_EDGE ( 'NONE', *, *, #4337, .T. ) ;
#14614=DIRECTION ( 'NONE',  ( 0.000000000000000000, 0.000000000000000000, 1.000000000000000000 ) ) ;
#14616=ADVANCED_FACE ( 'NONE', ( #7446 ), #4717, .T. ) ;
#14617=CARTESIAN_POINT ( 'NONE',  ( -66.39376235201207521, 88.50596986196454452, -15.00000000000001243 ) ) ;
#14618=ORIENTED_EDGE ( 'NONE', *, *, #14538, .T. ) ;
#14627=CYLINDRICAL_SURFACE ( 'NONE', #7866, 4.600000000000006750 ) ;
#14635=DIRECTION ( 'NONE',  ( 1.000000000000000000, 0.000000000000000000, 3.771137991253928573E-16 ) ) ;
#14640=DIRECTION ( 'NONE',  ( -1.000000000000000000, 3.016910393003142859E-15, 0.000000000000000000 ) ) ;
#14642=EDGE_CURVE ( 'NONE', #14698, #16861, #4379, .T. ) ;
#14643=DIRECTION ( 'NONE',  ( 0.000000000000000000, 0.000000000000000000, 1.000000000000000000 ) ) ;
#14644=EDGE_CURVE ( 'NONE', #13790, #16158, #11847, .T. ) ;
#14647=EDGE_LOOP ( 'NONE', ( #3257, #973, #11928, #11626 ) ) ;
#14655=LINE ( 'NONE', #1844, #18086 ) ;
#14673=CIRCLE ( 'NONE', #1548, 4.599999999999999645 ) ;
#14685=CARTESIAN_POINT ( 'NONE',  ( -47.59681378869034774, 80.34130291867735707, -15.00000000000001421 ) ) ;
#14686=ORIENTED_EDGE ( 'NONE', *, *, #16444, .T. ) ;
#14687=AXIS2_PLACEMENT_3D ( 'NONE', #16334, #14925, #10826 ) ;
#14690=CARTESIAN_POINT ( 'NONE',  ( -49.65031598894605480, 92.07579602767992810, -15.00000000000001421 ) ) ;
#14694=DIRECTION ( 'NONE',  ( 1.000000000000000000, 0.000000000000000000, 5.077734830647299712E-16 ) ) ;
#14698=VERTEX_POINT ( 'NONE', #8867 ) ;
#14699=AXIS2_PLACEMENT_3D ( 'NONE', #5469, #15398, #5366 ) ;
#14703=CARTESIAN_POINT ( 'NONE',  ( -67.00421887699711476, 86.78830982163884755, 15.00000000000006928 ) ) ;
#14710=VERTEX_POINT ( 'NONE', #15869 ) ;
#14711=AXIS2_PLACEMENT_3D ( 'NONE', #7129, #16850, #9757 ) ;
#14716=VECTOR ( 'NONE', #15204, 1000.000000000000000 ) ;
#14723=DIRECTION ( 'NONE',  ( 1.000000000000000000, 0.000000000000000000, 5.077734830647306615E-16 ) ) ;
#14735=VECTOR ( 'NONE', #5479, 1000.000000000000000 ) ;
#14738=DIRECTION ( 'NONE',  ( 0.000000000000000000, 0.000000000000000000, 1.000000000000000000 ) ) ;
#14742=FACE_OUTER_BOUND ( 'NONE', #1417, .T. ) ;
#14746=AXIS2_PLACEMENT_3D ( 'NONE', #15768, #17176, #5755 ) ;
#14753=AXIS2_PLACEMENT_3D ( 'NONE', #18322, #16907, #15502 ) ;
#14770=CIRCLE ( 'NONE', #18379, 4.599999999999992539 ) ;
#14777=CYLINDRICAL_SURFACE ( 'NONE', #5726, 4.600000000000006750 ) ;
#14778=ORIENTED_EDGE ( 'NONE', *, *, #150, .T. ) ;
#14781=CARTESIAN_POINT ( 'NONE',  ( -62.30871503255384170, 95.58244595420320877, -15.00000000000001421 ) ) ;
#14785=CIRCLE ( 'NONE', #5817, 12.49999999999999112 ) ;
#14786=DIRECTION ( 'NONE',  ( 1.000000000000000000, 0.000000000000000000, 3.771137991253923150E-16 ) ) ;
#14789=ORIENTED_EDGE ( 'NONE', *, *, #18306, .T. ) ;
#14793=CARTESIAN_POINT ( 'NONE',  ( -56.59294758719027385, 94.46597735006069740, 15.00000000000006928 ) ) ;
#14796=AXIS2_PLACEMENT_3D ( 'NONE', #10825, #5107, #9429 ) ;
#14798=ORIENTED_EDGE ( 'NONE', *, *, #1933, .F. ) ;
#14799=CARTESIAN_POINT ( 'NONE',  ( -57.08002265617300708, 84.22855780814606419, -167.1454815528550739 ) ) ;
#14800=CYLINDRICAL_SURFACE ( 'NONE', #11419, 4.600000000000006750 ) ;
#14811=ORIENTED_EDGE ( 'NONE', *, *, #14967, .T. ) ;
#14814=EDGE_LOOP ( 'NONE', ( #1998, #1517, #16483, #4349 ) ) ;
#14816=CARTESIAN_POINT ( 'NONE',  ( -47.80867013224673912, 89.78028827820993740, 15.00000000000006928 ) ) ;
#14818=DIRECTION ( 'NONE',  ( -5.204170427930409450E-16, 0.000000000000000000, 1.000000000000000000 ) ) ;
#14827=ORIENTED_EDGE ( 'NONE', *, *, #11507, .F. ) ;
#14828=FACE_OUTER_BOUND ( 'NONE', #3029, .T. ) ;
#14836=ORIENTED_EDGE ( 'NONE', *, *, #10179, .F. ) ;
#14839=DIRECTION ( 'NONE',  ( 1.156482317317869999E-16, 0.000000000000000000, 1.000000000000000000 ) ) ;
#14847=EDGE_CURVE ( 'NONE', #4088, #16289, #2358, .T. ) ;
#14848=FACE_OUTER_BOUND ( 'NONE', #5482, .T. ) ;
#14851=ORIENTED_EDGE ( 'NONE', *, *, #5626, .F. ) ;
#14852=FACE_OUTER_BOUND ( 'NONE', #3323, .T. ) ;
#14854=ORIENTED_EDGE ( 'NONE', *, *, #16113, .T. ) ;
#14861=CYLINDRICAL_SURFACE ( 'NONE', #1262, 4.600000000000013856 ) ;
#14862=EDGE_LOOP ( 'NONE', ( #8434, #14410, #11650, #6505 ) ) ;
#14867=EDGE_CURVE ( 'NONE', #16085, #16195, #3803, .T. ) ;
#14869=DIRECTION ( 'NONE',  ( 0.000000000000000000, 0.000000000000000000, 1.000000000000000000 ) ) ;
#14873=EDGE_CURVE ( 'NONE', #10224, #9544, #5485, .T. ) ;
#14879=DIRECTION ( 'NONE',  ( -1.000000000000000000, 6.033820786006295184E-15, 0.000000000000000000 ) ) ;
#14887=DIRECTION ( 'NONE',  ( 1.000000000000000000, 0.000000000000000000, 0.000000000000000000 ) ) ;
#14888=DIRECTION ( 'NONE',  ( -1.000000000000000000, -3.016910393003147592E-15, 0.000000000000000000 ) ) ;
#14891=ORIENTED_EDGE ( 'NONE', *, *, #16480, .T. ) ;
#14896=AXIS2_PLACEMENT_3D ( 'NONE', #12938, #18460, #7130 ) ;
#14901=ORIENTED_EDGE ( 'NONE', *, *, #10429, .T. ) ;
#14903=VERTEX_POINT ( 'NONE', #1291 ) ;
#14908=CARTESIAN_POINT ( 'NONE',  ( -57.08002265617300708, 84.22855780814606419, 15.00000000000006928 ) ) ;
#14914=CARTESIAN_POINT ( 'NONE',  ( -63.37199650155329778, 75.44273092821040905, 15.00000000000006928 ) ) ;
#14917=CYLINDRICAL_SURFACE ( 'NONE', #5832, 12.50000000000000355 ) ;
#14919=DIRECTION ( 'NONE',  ( -1.000000000000000000, -3.774758283725530975E-14, 1.387778780781445182E-16 ) ) ;
#14920=FACE_OUTER_BOUND ( 'NONE', #6371, .T. ) ;
#14925=DIRECTION ( 'NONE',  ( -5.204170427930409450E-16, 0.000000000000000000, 1.000000000000000000 ) ) ;
#14934=VERTEX_POINT ( 'NONE', #15412 ) ;
#14939=ORIENTED_EDGE ( 'NONE', *, *, #2655, .T. ) ;
#14948=DIRECTION ( 'NONE',  ( 1.000000000000000000, 0.000000000000000000, 0.000000000000000000 ) ) ;
#14954=EDGE_CURVE ( 'NONE', #15261, #768, #8095, .T. ) ;
#14955=CIRCLE ( 'NONE', #3028, 10.24900000000000055 ) ;
#14958=DIRECTION ( 'NONE',  ( 1.000000000000000000, 0.000000000000000000, 0.000000000000000000 ) ) ;
#14959=VERTEX_POINT ( 'NONE', #16610 ) ;
#14966=CARTESIAN_POINT ( 'NONE',  ( -57.08002265617300708, 84.22855780814606419, 15.00000000000006928 ) ) ;
#14967=EDGE_CURVE ( 'NONE', #4389, #9420, #9704, .T. ) ;
#14968=CYLINDRICAL_SURFACE ( 'NONE', #10005, 10.24900000000000766 ) ;
#14970=EDGE_CURVE ( 'NONE', #3203, #3299, #12716, .T. ) ;
#14981=VERTEX_POINT ( 'NONE', #7262 ) ;
#14985=ADVANCED_FACE ( 'NONE', ( #17256 ), #237, .T. ) ;
#14988=VERTEX_POINT ( 'NONE', #61 ) ;
#14990=ORIENTED_EDGE ( 'NONE', *, *, #972, .T. ) ;
#14999=ORIENTED_EDGE ( 'NONE', *, *, #10856, .F. ) ;
#15003=DIRECTION ( 'NONE',  ( -1.000000000000000000, 0.000000000000000000, 1.387778780781446662E-16 ) ) ;
#15005=ORIENTED_EDGE ( 'NONE', *, *, #6165, .F. ) ;
#15007=CIRCLE ( 'NONE', #83, 4.599999999999999645 ) ;
#15037=ORIENTED_EDGE ( 'NONE', *, *, #3103, .F. ) ;
#15039=EDGE_CURVE ( 'NONE', #583, #12181, #14345, .T. ) ;
#15044=DIRECTION ( 'NONE',  ( -5.204170427930409450E-16, 0.000000000000000000, 1.000000000000000000 ) ) ;
#15047=SHAPE_REPRESENTATION ( 'Drive Gear', ( #16217 ), #9669 ) ;
#15054=ORIENTED_EDGE ( 'NONE', *, *, #4698, .F. ) ;
#15057=VERTEX_POINT ( 'NONE', #8662 ) ;
#15073=CARTESIAN_POINT ( 'NONE',  ( -57.35243698450333483, 71.73152654333280509, -15.00000000000001421 ) ) ;
#15075=AXIS2_PLACEMENT_3D ( 'NONE', #8776, #1473, #8866 ) ;
#15076=DIRECTION ( 'NONE',  ( 1.000000000000000000, 0.000000000000000000, 3.771137991253928573E-16 ) ) ;
#15078=CARTESIAN_POINT ( 'NONE',  ( -69.52933024547458274, 85.35316464920589397, 15.00000000000006750 ) ) ;
#15095=EDGE_CURVE ( 'NONE', #8377, #3838, #11645, .T. ) ;
#15098=EDGE_CURVE ( 'NONE', #4520, #11983, #7360, .T. ) ;
#15103=EDGE_CURVE ( 'NONE', #5567, #5776, #12861, .T. ) ;
#15107=DIRECTION ( 'NONE',  ( 1.156482317317869999E-16, 0.000000000000000000, 1.000000000000000000 ) ) ;
#15115=FACE_OUTER_BOUND ( 'NONE', #14647, .T. ) ;
#15125=CARTESIAN_POINT ( 'NONE',  ( -47.27059076829218043, 81.25920652595885940, -167.1454815528550739 ) ) ;
#15130=VERTEX_POINT ( 'NONE', #9282 ) ;
#15134=ORIENTED_EDGE ( 'NONE', *, *, #3879, .F. ) ;
#15137=DIRECTION ( 'NONE',  ( -5.204170427930409450E-16, 0.000000000000000000, 1.000000000000000000 ) ) ;
#15139=CARTESIAN_POINT ( 'NONE',  ( -66.56323152365561668, 80.34130291867722917, -167.1454815528550739 ) ) ;
#15143=ORIENTED_EDGE ( 'NONE', *, *, #17838, .F. ) ;
#15147=ORIENTED_EDGE ( 'NONE', *, *, #3300, .F. ) ;
#15148=EDGE_CURVE ( 'NONE', #8149, #13790, #6553, .T. ) ;
#15150=FACE_OUTER_BOUND ( 'NONE', #1795, .T. ) ;
#15153=EDGE_LOOP ( 'NONE', ( #12697, #14541, #9696, #14520 ) ) ;
#15154=DIRECTION ( 'NONE',  ( -1.000000000000000000, 0.000000000000000000, 1.692578276882434470E-16 ) ) ;
#15155=CARTESIAN_POINT ( 'NONE',  ( -57.08002265617300708, 84.22855780814606419, 15.00000000000006928 ) ) ;
#15163=CARTESIAN_POINT ( 'NONE',  ( -56.80760832784252301, 71.73152654333280509, 15.00000000000006928 ) ) ;
#15180=CARTESIAN_POINT ( 'NONE',  ( -57.08002265617300708, 84.22855780814606419, -167.1454815528550739 ) ) ;
#15184=DIRECTION ( 'NONE',  ( 1.000000000000000000, 0.000000000000000000, 5.077734830647302671E-16 ) ) ;
#15186=DIRECTION ( 'NONE',  ( 1.000000000000000000, 0.000000000000000000, 0.000000000000000000 ) ) ;
#15188=DIRECTION ( 'NONE',  ( 1.000000000000000000, 0.000000000000000000, 3.771137991253923150E-16 ) ) ;
#15198=DIRECTION ( 'NONE',  ( -5.204170427930409450E-16, 0.000000000000000000, 1.000000000000000000 ) ) ;
#15204=DIRECTION ( 'NONE',  ( 0.000000000000000000, 0.000000000000000000, 1.000000000000000000 ) ) ;
#15210=AXIS2_PLACEMENT_3D ( 'NONE', #17352, #1832, #518 ) ;
#15211=CYLINDRICAL_SURFACE ( 'NONE', #8839, 4.600000000000006750 ) ;
#15215=DIRECTION ( 'NONE',  ( 0.000000000000000000, 0.000000000000000000, 1.000000000000000000 ) ) ;
#15220=ORIENTED_EDGE ( 'NONE', *, *, #5730, .T. ) ;
#15221=EDGE_CURVE ( 'NONE', #1636, #1562, #12182, .T. ) ;
#15230=VERTEX_POINT ( 'NONE', #774 ) ;
#15235=CYLINDRICAL_SURFACE ( 'NONE', #3738, 4.599999999999999645 ) ;
#15239=AXIS2_PLACEMENT_3D ( 'NONE', #9947, #11271, #16957 ) ;
#15247=VERTEX_POINT ( 'NONE', #17971 ) ;
#15248=ORIENTED_EDGE ( 'NONE', *, *, #13705, .F. ) ;
#15249=CIRCLE ( 'NONE', #11960, 4.599999999999992539 ) ;
#15260=CARTESIAN_POINT ( 'NONE',  ( -67.13262496892538422, 91.65790412808873100, 15.00000000000006928 ) ) ;
#15261=VERTEX_POINT ( 'NONE', #2733 ) ;
#15265=ORIENTED_EDGE ( 'NONE', *, *, #3196, .F. ) ;
#15280=ORIENTED_EDGE ( 'NONE', *, *, #3878, .T. ) ;
#15287=DIRECTION ( 'NONE',  ( 0.000000000000000000, 0.000000000000000000, 1.000000000000000000 ) ) ;
#15297=ADVANCED_FACE ( 'NONE', ( #4227 ), #1513, .T. ) ;
#15303=CARTESIAN_POINT ( 'NONE',  ( -45.21333244822126574, 88.15687341518456321, -167.1454815528550739 ) ) ;
#15307=DIRECTION ( 'NONE',  ( 1.000000000000000000, 0.000000000000000000, 0.000000000000000000 ) ) ;
#15308=VECTOR ( 'NONE', #18199, 1000.000000000000000 ) ;
#15310=CARTESIAN_POINT ( 'NONE',  ( -46.36441787118067026, 82.83016482797245317, -15.00000000000001421 ) ) ;
#15311=DIRECTION ( 'NONE',  ( -1.000000000000000000, 0.000000000000000000, 1.692578276882434470E-16 ) ) ;
#15317=CIRCLE ( 'NONE', #11155, 4.599999999999999645 ) ;
#15319=EDGE_CURVE ( 'NONE', #626, #11065, #14044, .T. ) ;
#15321=VERTEX_POINT ( 'NONE', #14250 ) ;
#15323=ORIENTED_EDGE ( 'NONE', *, *, #989, .F. ) ;
#15327=AXIS2_PLACEMENT_3D ( 'NONE', #925, #10944, #17848 ) ;
#15335=AXIS2_PLACEMENT_3D ( 'NONE', #13486, #17782, #7685 ) ;
#15336=CIRCLE ( 'NONE', #9066, 12.50000000000000355 ) ;
#15337=EDGE_CURVE ( 'NONE', #9366, #8099, #1343, .T. ) ;
#15349=EDGE_CURVE ( 'NONE', #14316, #14366, #9654, .T. ) ;
#15366=VERTEX_POINT ( 'NONE', #4054 ) ;
#15374=EDGE_LOOP ( 'NONE', ( #2616, #7424, #13913, #2849 ) ) ;
#15383=VECTOR ( 'NONE', #15564, 1000.000000000000000 ) ;
#15385=CARTESIAN_POINT ( 'NONE',  ( -49.75809927370887920, 76.28065702765852052, 15.00000000000006928 ) ) ;
#15396=ORIENTED_EDGE ( 'NONE', *, *, #6169, .T. ) ;
#15398=DIRECTION ( 'NONE',  ( -5.204170427930409450E-16, 0.000000000000000000, 1.000000000000000000 ) ) ;
#15412=CARTESIAN_POINT ( 'NONE',  ( -53.84898691462515785, 93.95493478196527803, 15.00000000000006928 ) ) ;
#15413=DIRECTION ( 'NONE',  ( 0.000000000000000000, 0.000000000000000000, 1.000000000000000000 ) ) ;
#15414=CARTESIAN_POINT ( 'NONE',  ( -66.35137518009933899, 89.78028827820979529, -15.00000000000001421 ) ) ;
#15419=FACE_OUTER_BOUND ( 'NONE', #11758, .T. ) ;
#15420=AXIS2_PLACEMENT_3D ( 'NONE', #15727, #265, #4557 ) ;
#15428=ORIENTED_EDGE ( 'NONE', *, *, #3079, .T. ) ;
#15429=ORIENTED_EDGE ( 'NONE', *, *, #809, .F. ) ;
#15434=LINE ( 'NONE', #15139, #12977 ) ;
#15438=DIRECTION ( 'NONE',  ( 0.000000000000000000, 0.000000000000000000, 1.000000000000000000 ) ) ;
#15442=EDGE_CURVE ( 'NONE', #16069, #5776, #18367, .T. ) ;
#15468=VERTEX_POINT ( 'NONE', #7669 ) ;
#15480=ORIENTED_EDGE ( 'NONE', *, *, #3534, .F. ) ;
#15486=DIRECTION ( 'NONE',  ( -1.000000000000000000, -3.016910393003138520E-15, 0.000000000000000000 ) ) ;
#15497=DIRECTION ( 'NONE',  ( -1.000000000000000000, 0.000000000000000000, 1.387778780781445182E-16 ) ) ;
#15499=ORIENTED_EDGE ( 'NONE', *, *, #17838, .T. ) ;
#15502=DIRECTION ( 'NONE',  ( 1.000000000000000000, 0.000000000000000000, 0.000000000000000000 ) ) ;
#15503=AXIS2_PLACEMENT_3D ( 'NONE', #7767, #9000, #14786 ) ;
#15510=DIRECTION ( 'NONE',  ( 0.000000000000000000, 0.000000000000000000, 1.000000000000000000 ) ) ;
#15513=VECTOR ( 'NONE', #18124, 1000.000000000000000 ) ;
#15517=CARTESIAN_POINT ( 'NONE',  ( -64.89435165812551531, 90.86016871721213306, -167.1454815528550739 ) ) ;
#15518=CARTESIAN_POINT ( 'NONE',  ( -44.59353464447068660, 84.80960611389554060, -167.1454815528550739 ) ) ;
#15526=ORIENTED_EDGE ( 'NONE', *, *, #15442, .F. ) ;
#15528=DIRECTION ( 'NONE',  ( 0.000000000000000000, 0.000000000000000000, 1.000000000000000000 ) ) ;
#15530=ORIENTED_EDGE ( 'NONE', *, *, #952, .T. ) ;
#15534=EDGE_LOOP ( 'NONE', ( #16545, #15933, #11617, #8043 ) ) ;
#15535=ORIENTED_EDGE ( 'NONE', *, *, #10802, .F. ) ;
#15540=LINE ( 'NONE', #1600, #3256 ) ;
#15549=DIRECTION ( 'NONE',  ( 1.156482317317869999E-16, 0.000000000000000000, 1.000000000000000000 ) ) ;
#15558=VECTOR ( 'NONE', #6450, 1000.000000000000000 ) ;
#15564=DIRECTION ( 'NONE',  ( 0.000000000000000000, 0.000000000000000000, 1.000000000000000000 ) ) ;
#15565=ADVANCED_FACE ( 'NONE', ( #16074 ), #753, .T. ) ;
#15570=AXIS2_PLACEMENT_3D ( 'NONE', #18291, #2475, #8077 ) ;
#15571=ORIENTED_EDGE ( 'NONE', *, *, #2255, .F. ) ;
#15576=CARTESIAN_POINT ( 'NONE',  ( -57.08002265617300708, 84.22855780814606419, -15.00000000000001421 ) ) ;
#15584=DIRECTION ( 'NONE',  ( 1.000000000000000000, 0.000000000000000000, 5.551115123125780730E-16 ) ) ;
#15595=FACE_OUTER_BOUND ( 'NONE', #1726, .T. ) ;
#15613=DIRECTION ( 'NONE',  ( 0.000000000000000000, 0.000000000000000000, 1.000000000000000000 ) ) ;
#15615=ORIENTED_EDGE ( 'NONE', *, *, #9637, .F. ) ;
#15616=VERTEX_POINT ( 'NONE', #3742 ) ;
#15625=VERTEX_POINT ( 'NONE', #10747 ) ;
#15630=ORIENTED_EDGE ( 'NONE', *, *, #13474, .T. ) ;
#15637=CIRCLE ( 'NONE', #14141, 4.599999999999999645 ) ;
#15649=CARTESIAN_POINT ( 'NONE',  ( -56.41614838398844256, 95.01461175692088545, -167.1454815528550739 ) ) ;
#15652=CARTESIAN_POINT ( 'NONE',  ( -57.08002265617300708, 84.22855780814606419, -167.1454815528550739 ) ) ;
#15653=ORIENTED_EDGE ( 'NONE', *, *, #13989, .F. ) ;
#15655=ORIENTED_EDGE ( 'NONE', *, *, #14867, .T. ) ;
#15659=DIRECTION ( 'NONE',  ( 1.000000000000000000, 0.000000000000000000, 5.551115123125780730E-16 ) ) ;
#15677=ORIENTED_EDGE ( 'NONE', *, *, #6982, .F. ) ;
#15692=ADVANCED_FACE ( 'NONE', ( #8029 ), #6532, .T. ) ;
#15694=DIRECTION ( 'NONE',  ( 0.000000000000000000, 0.000000000000000000, 1.000000000000000000 ) ) ;
#15695=FACE_OUTER_BOUND ( 'NONE', #3125, .T. ) ;
#15704=CARTESIAN_POINT ( 'NONE',  ( -56.26901274438541378, 73.45256821284058901, 15.00000000000006928 ) ) ;
#15708=CIRCLE ( 'NONE', #7619, 12.49999999999999112 ) ;
#15714=FACE_OUTER_BOUND ( 'NONE', #18062, .T. ) ;
#15715=DIRECTION ( 'NONE',  ( -5.204170427930409450E-16, 0.000000000000000000, 1.000000000000000000 ) ) ;
#15720=VERTEX_POINT ( 'NONE', #9632 ) ;
#15727=CARTESIAN_POINT ( 'NONE',  ( -59.35080917176598092, 94.79374675277695417, -167.1454815528550739 ) ) ;
#15733=CARTESIAN_POINT ( 'NONE',  ( -47.80867013224673912, 89.78028827820993740, -167.1454815528550739 ) ) ;
#15741=CARTESIAN_POINT ( 'NONE',  ( -56.59294758719027385, 94.46597735006069740, -15.00000000000001421 ) ) ;
#15742=ORIENTED_EDGE ( 'NONE', *, *, #13616, .F. ) ;
#15746=LINE ( 'NONE', #4412, #9565 ) ;
#15748=DIRECTION ( 'NONE',  ( 1.000000000000000000, 0.000000000000000000, 3.771137991253934490E-16 ) ) ;
#15749=ORIENTED_EDGE ( 'NONE', *, *, #8914, .T. ) ;
#15756=DIRECTION ( 'NONE',  ( 0.000000000000000000, 0.000000000000000000, 1.000000000000000000 ) ) ;
#15758=DIRECTION ( 'NONE',  ( -1.000000000000000000, 1.099120794378904723E-13, 1.387778780781445182E-16 ) ) ;
#15765=ORIENTED_EDGE ( 'NONE', *, *, #14433, .T. ) ;
#15767=ORIENTED_EDGE ( 'NONE', *, *, #5612, .F. ) ;
#15768=CARTESIAN_POINT ( 'NONE',  ( -57.08002265617300708, 84.22855780814606419, -167.1454815528550739 ) ) ;
#15772=CARTESIAN_POINT ( 'NONE',  ( -57.08002265617300708, 84.22855780814606419, 15.00000000000006928 ) ) ;
#15777=FACE_OUTER_BOUND ( 'NONE', #3417, .T. ) ;
#15783=CARTESIAN_POINT ( 'NONE',  ( -66.39376235201207521, 88.50596986196454452, -167.1454815528550739 ) ) ;
#15786=CYLINDRICAL_SURFACE ( 'NONE', #2401, 12.49999999999999112 ) ;
#15790=EDGE_CURVE ( 'NONE', #17935, #9354, #7188, .T. ) ;
#15793=FACE_OUTER_BOUND ( 'NONE', #17179, .T. ) ;
#15812=CIRCLE ( 'NONE', #7438, 4.600000000000006750 ) ;
#15816=CARTESIAN_POINT ( 'NONE',  ( -46.69442755757756203, 81.24207102880484399, 15.00000000000009592 ) ) ;
#15827=DIRECTION ( 'NONE',  ( 1.000000000000000000, 0.000000000000000000, 3.771137991253923150E-16 ) ) ;
#15834=CARTESIAN_POINT ( 'NONE',  ( -47.19781944808393348, 88.60139997190906058, 15.00000000000009592 ) ) ;
#15842=DIRECTION ( 'NONE',  ( -1.000000000000000000, 0.000000000000000000, 0.000000000000000000 ) ) ;
#15855=FACE_OUTER_BOUND ( 'NONE', #30, .T. ) ;
#15857=AXIS2_PLACEMENT_3D ( 'NONE', #9800, #16802, #14111 ) ;
#15858=DIRECTION ( 'NONE',  ( 0.000000000000000000, 0.000000000000000000, 1.000000000000000000 ) ) ;
#15863=CARTESIAN_POINT ( 'NONE',  ( -46.27380910617147691, 84.15481808402802244, -167.1454815528550739 ) ) ;
#15869=CARTESIAN_POINT ( 'NONE',  ( -53.97067643794850511, 72.12145385653101926, 15.00000000000006928 ) ) ;
#15875=DIRECTION ( 'NONE',  ( 1.000000000000000000, 0.000000000000000000, 0.000000000000000000 ) ) ;
#15878=CARTESIAN_POINT ( 'NONE',  ( -57.08002265617300708, 84.22855780814606419, 15.00000000000006928 ) ) ;
#15880=EDGE_LOOP ( 'NONE', ( #2262, #1421, #2417, #5606 ) ) ;
#15885=FACE_OUTER_BOUND ( 'NONE', #13128, .T. ) ;
#15895=DIRECTION ( 'NONE',  ( 1.156482317317869999E-16, 0.000000000000000000, 1.000000000000000000 ) ) ;
#15902=EDGE_CURVE ( 'NONE', #10995, #5674, #7555, .T. ) ;
#15913=DIRECTION ( 'NONE',  ( 1.000000000000000000, 0.000000000000000000, 3.771137991253928573E-16 ) ) ;
#15933=ORIENTED_EDGE ( 'NONE', *, *, #10085, .T. ) ;
#15942=AXIS2_PLACEMENT_3D ( 'NONE', #2360, #8068, #5455 ) ;
#15953=CARTESIAN_POINT ( 'NONE',  ( -69.37109144396066540, 81.95267818613797317, 15.00000000000006928 ) ) ;
#15956=ADVANCED_FACE ( 'NONE', ( #7378 ), #10274, .T. ) ;
#15959=DIRECTION ( 'NONE',  ( 1.156482317317869999E-16, 0.000000000000000000, 1.000000000000000000 ) ) ;
#15960=EDGE_LOOP ( 'NONE', ( #11779, #16688, #13166, #40 ) ) ;
#15962=DIRECTION ( 'NONE',  ( 0.000000000000000000, 0.000000000000000000, 1.000000000000000000 ) ) ;
#15964=CARTESIAN_POINT ( 'NONE',  ( -67.00421887699711476, 86.78830982163884755, -167.1454815528550739 ) ) ;
#15976=AXIS2_PLACEMENT_3D ( 'NONE', #14908, #17625, #16223 ) ;
#15977=DIRECTION ( 'NONE',  ( 0.000000000000000000, 0.000000000000000000, 1.000000000000000000 ) ) ;
#15982=CARTESIAN_POINT ( 'NONE',  ( -46.65463807863145007, 87.07303407725225952, -167.1454815528550739 ) ) ;
#15991=CIRCLE ( 'NONE', #4062, 10.24900000000000055 ) ;
#15992=AXIS2_PLACEMENT_3D ( 'NONE', #17207, #4391, #10099 ) ;
#16009=CARTESIAN_POINT ( 'NONE',  ( -47.76628296033400289, 88.50596986196467242, 15.00000000000006928 ) ) ;
#16012=VERTEX_POINT ( 'NONE', #10822 ) ;
#16016=DIRECTION ( 'NONE',  ( 1.156482317317869999E-16, 0.000000000000000000, 1.000000000000000000 ) ) ;
#16019=ADVANCED_FACE ( 'NONE', ( #4930 ), #6317, .T. ) ;
#16027=DIRECTION ( 'NONE',  ( 1.000000000000000000, 0.000000000000000000, 5.077734830647295768E-16 ) ) ;
#16028=ORIENTED_EDGE ( 'NONE', *, *, #4981, .T. ) ;
#16037=DIRECTION ( 'NONE',  ( 0.000000000000000000, 0.000000000000000000, 1.000000000000000000 ) ) ;
#16041=DIRECTION ( 'NONE',  ( 1.000000000000000000, 0.000000000000000000, 0.000000000000000000 ) ) ;
#16042=CARTESIAN_POINT ( 'NONE',  ( -48.65098454476478196, 77.46608744949921288, -15.00000000000001421 ) ) ;
#16051=CARTESIAN_POINT ( 'NONE',  ( -52.04298920050707977, 93.78931001713317528, -167.1454815528550739 ) ) ;
#16064=CARTESIAN_POINT ( 'NONE',  ( -53.29103256796045684, 73.45256821284057480, -15.00000000000001421 ) ) ;
#16068=AXIS2_PLACEMENT_3D ( 'NONE', #4501, #1524, #7234 ) ;
#16069=VERTEX_POINT ( 'NONE', #4827 ) ;
#16070=CARTESIAN_POINT ( 'NONE',  ( -57.08002265617300708, 84.22855780814606419, -15.00000000000001421 ) ) ;
#16071=DIRECTION ( 'NONE',  ( 1.000000000000000000, 0.000000000000000000, 3.771137991253923150E-16 ) ) ;
#16073=DIRECTION ( 'NONE',  ( -1.000000000000000000, -3.016910393003138520E-15, 0.000000000000000000 ) ) ;
#16074=FACE_OUTER_BOUND ( 'NONE', #18152, .T. ) ;
#16085=VERTEX_POINT ( 'NONE', #10930 ) ;
#16091=ORIENTED_EDGE ( 'NONE', *, *, #3459, .T. ) ;
#16094=ORIENTED_EDGE ( 'NONE', *, *, #17886, .F. ) ;
#16102=EDGE_CURVE ( 'NONE', #12783, #9284, #10724, .T. ) ;
#16107=ADVANCED_FACE ( 'NONE', ( #13819 ), #9510, .T. ) ;
#16113=EDGE_CURVE ( 'NONE', #12461, #10547, #3586, .T. ) ;
#16119=AXIS2_PLACEMENT_3D ( 'NONE', #8728, #209, #8634 ) ;
#16135=AXIS2_PLACEMENT_3D ( 'NONE', #75, #7182, #1206 ) ;
#16137=CARTESIAN_POINT ( 'NONE',  ( -66.02736529514692165, 75.49957964911740760, -15.00000000000001243 ) ) ;
#16141=CARTESIAN_POINT ( 'NONE',  ( -63.37199650155329778, 75.44273092821040905, -167.1454815528550739 ) ) ;
#16147=CARTESIAN_POINT ( 'NONE',  ( -55.20348911625212907, 74.15281352429526862, -167.1454815528550739 ) ) ;
#16150=CIRCLE ( 'NONE', #10785, 4.599999999999992539 ) ;
#16158=VERTEX_POINT ( 'NONE', #18221 ) ;
#16159=EDGE_LOOP ( 'NONE', ( #7541, #17750, #14778, #12866 ) ) ;
#16160=CIRCLE ( 'NONE', #8109, 12.50000000000001776 ) ;
#16162=CARTESIAN_POINT ( 'NONE',  ( -57.08002265617300708, 84.22855780814606419, 15.00000000000006928 ) ) ;
#16167=CARTESIAN_POINT ( 'NONE',  ( -61.60537251683745552, 75.03273214436880778, 15.00000000000006928 ) ) ;
#16168=ORIENTED_EDGE ( 'NONE', *, *, #14642, .T. ) ;
#16170=CARTESIAN_POINT ( 'NONE',  ( -57.08002265617300708, 84.22855780814606419, -167.1454815528550739 ) ) ;
#16171=CIRCLE ( 'NONE', #14407, 4.600000000000006750 ) ;
#16174=ORIENTED_EDGE ( 'NONE', *, *, #6060, .T. ) ;
#16178=VECTOR ( 'NONE', #13182, 1000.000000000000000 ) ;
#16180=ORIENTED_EDGE ( 'NONE', *, *, #3312, .F. ) ;
#16183=CARTESIAN_POINT ( 'NONE',  ( -46.10942163047475617, 78.23723799236688592, 15.00000000000006928 ) ) ;
#16187=AXIS2_PLACEMENT_3D ( 'NONE', #2104, #15107, #710 ) ;
#16195=VERTEX_POINT ( 'NONE', #5582 ) ;
#16197=ORIENTED_EDGE ( 'NONE', *, *, #4933, .F. ) ;
#16205=AXIS2_PLACEMENT_3D ( 'NONE', #13947, #1131, #5237 ) ;
#16209=CIRCLE ( 'NONE', #8168, 12.49999999999999112 ) ;
#16217=AXIS2_PLACEMENT_3D ( 'NONE', #5781, #6037, #8961 ) ;
#16223=DIRECTION ( 'NONE',  ( 1.000000000000000000, 0.000000000000000000, 5.551115123125777772E-16 ) ) ;
#16229=EDGE_LOOP ( 'NONE', ( #370, #16549, #11195, #8053 ) ) ;
#16231=AXIS2_PLACEMENT_3D ( 'NONE', #3509, #9224, #2112 ) ;
#16239=DIRECTION ( 'NONE',  ( 0.000000000000000000, 0.000000000000000000, 1.000000000000000000 ) ) ;
#16240=CARTESIAN_POINT ( 'NONE',  ( -50.24148097183213935, 76.59466308582166505, -15.00000000000001421 ) ) ;
#16242=ORIENTED_EDGE ( 'NONE', *, *, #7665, .T. ) ;
#16243=CARTESIAN_POINT ( 'NONE',  ( -48.21445538031289857, 89.37090336996882911, -167.1454815528550739 ) ) ;
#16248=EDGE_CURVE ( 'NONE', #10547, #9500, #14374, .T. ) ;
#16255=DIRECTION ( 'NONE',  ( 0.000000000000000000, 0.000000000000000000, 1.000000000000000000 ) ) ;
#16256=LINE ( 'NONE', #17756, #12269 ) ;
#16258=EDGE_CURVE ( 'NONE', #14160, #17041, #1529, .T. ) ;
#16261=ORIENTED_EDGE ( 'NONE', *, *, #1720, .T. ) ;
#16265=AXIS2_PLACEMENT_3D ( 'NONE', #14379, #17193, #4377 ) ;
#16268=CIRCLE ( 'NONE', #4899, 10.24900000000000055 ) ;
#16273=CARTESIAN_POINT ( 'NONE',  ( -51.81614838398844824, 95.01461175692088545, 15.00000000000007105 ) ) ;
#16280=CIRCLE ( 'NONE', #8227, 12.49999999999999112 ) ;
#16282=AXIS2_PLACEMENT_3D ( 'NONE', #6313, #4924, #7725 ) ;
#16284=ORIENTED_EDGE ( 'NONE', *, *, #5925, .T. ) ;
#16287=DIRECTION ( 'NONE',  ( 1.000000000000000000, 0.000000000000000000, 0.000000000000000000 ) ) ;
#16288=CARTESIAN_POINT ( 'NONE',  ( -57.08002265617300708, 84.22855780814606419, 15.00000000000006928 ) ) ;
#16289=VERTEX_POINT ( 'NONE', #7267 ) ;
#16292=AXIS2_PLACEMENT_3D ( 'NONE', #18441, #17015, #7198 ) ;
#16297=CARTESIAN_POINT ( 'NONE',  ( -48.99724571598702738, 77.92691374209489652, -15.00000000000001421 ) ) ;
#16299=EDGE_LOOP ( 'NONE', ( #6332, #4802, #17826, #2005 ) ) ;
#16303=ORIENTED_EDGE ( 'NONE', *, *, #8719, .F. ) ;
#16310=ORIENTED_EDGE ( 'NONE', *, *, #10593, .T. ) ;
#16327=DIRECTION ( 'NONE',  ( 0.000000000000000000, 0.000000000000000000, 1.000000000000000000 ) ) ;
#16334=CARTESIAN_POINT ( 'NONE',  ( -64.40194603863702127, 76.28065702765842104, 15.00000000000006928 ) ) ;
#16337=LINE ( 'NONE', #9335, #3723 ) ;
#16342=DIRECTION ( 'NONE',  ( -1.000000000000000000, -1.895687670108323806E-14, 1.692578276882432005E-16 ) ) ;
#16344=EDGE_CURVE ( 'NONE', #6741, #15230, #12904, .T. ) ;
#16347=ADVANCED_FACE ( 'NONE', ( #15777 ), #14471, .T. ) ;
#16351=CARTESIAN_POINT ( 'NONE',  ( -69.37109144396066540, 81.95267818613797317, -15.00000000000001421 ) ) ;
#16356=DIRECTION ( 'NONE',  ( -5.204170427930409450E-16, 0.000000000000000000, 1.000000000000000000 ) ) ;
#16374=DIRECTION ( 'NONE',  ( -1.000000000000000000, 0.000000000000000000, 1.692578276882434470E-16 ) ) ;
#16383=DIRECTION ( 'NONE',  ( -5.204170427930409450E-16, 0.000000000000000000, 1.000000000000000000 ) ) ;
#16403=AXIS2_PLACEMENT_3D ( 'NONE', #13677, #17788, #16374 ) ;
#16418=VERTEX_POINT ( 'NONE', #12023 ) ;
#16423=ORIENTED_EDGE ( 'NONE', *, *, #13813, .F. ) ;
#16432=AXIS2_PLACEMENT_3D ( 'NONE', #1861, #4840, #7386 ) ;
#16444=EDGE_CURVE ( 'NONE', #18394, #3838, #13481, .T. ) ;
#16446=CARTESIAN_POINT ( 'NONE',  ( -66.56323152365561668, 80.34130291867722917, 15.00000000000006928 ) ) ;
#16461=ORIENTED_EDGE ( 'NONE', *, *, #1720, .F. ) ;
#16469=CIRCLE ( 'NONE', #3929, 4.600000000000006750 ) ;
#16475=CARTESIAN_POINT ( 'NONE',  ( -57.08002265617300708, 84.22855780814606419, -15.00000000000001421 ) ) ;
#16477=CIRCLE ( 'NONE', #659, 7.500000000000000000 ) ;
#16480=EDGE_CURVE ( 'NONE', #11833, #10611, #16150, .T. ) ;
#16483=ORIENTED_EDGE ( 'NONE', *, *, #4473, .T. ) ;
#16488=AXIS2_PLACEMENT_3D ( 'NONE', #16042, #14558, #14640 ) ;
#16507=ORIENTED_EDGE ( 'NONE', *, *, #4456, .F. ) ;
#16512=CIRCLE ( 'NONE', #14711, 4.599999999999992539 ) ;
#16516=CIRCLE ( 'NONE', #7270, 10.24900000000000766 ) ;
#16518=CARTESIAN_POINT ( 'NONE',  ( -52.17699016282484337, 93.22868410554724505, 15.00000000000006928 ) ) ;
#16519=EDGE_LOOP ( 'NONE', ( #8954, #9272, #9767, #6890 ) ) ;
#16521=DIRECTION ( 'NONE',  ( 1.156482317317869999E-16, 0.000000000000000000, 1.000000000000000000 ) ) ;
#16525=DIRECTION ( 'NONE',  ( 0.000000000000000000, 0.000000000000000000, 1.000000000000000000 ) ) ;
#16533=CIRCLE ( 'NONE', #16839, 4.600000000000006750 ) ;
#16537=CARTESIAN_POINT ( 'NONE',  ( -57.08002265617300708, 84.22855780814606419, 15.00000000000006928 ) ) ;
#16542=DIRECTION ( 'NONE',  ( 1.000000000000000000, 0.000000000000000000, 0.000000000000000000 ) ) ;
#16545=ORIENTED_EDGE ( 'NONE', *, *, #3676, .F. ) ;
#16549=ORIENTED_EDGE ( 'NONE', *, *, #17503, .F. ) ;
#16552=DIRECTION ( 'NONE',  ( 1.000000000000000000, 0.000000000000000000, 5.551115123125784674E-16 ) ) ;
#16577=ORIENTED_EDGE ( 'NONE', *, *, #17697, .F. ) ;
#16581=EDGE_CURVE ( 'NONE', #16893, #2633, #1236, .T. ) ;
#16583=CIRCLE ( 'NONE', #8553, 12.50000000000000355 ) ;
#16590=ORIENTED_EDGE ( 'NONE', *, *, #9619, .T. ) ;
#16592=CARTESIAN_POINT ( 'NONE',  ( -57.08002265617300708, 84.22855780814606419, -15.00000000000001421 ) ) ;
#16593=CARTESIAN_POINT ( 'NONE',  ( -56.41614838398844256, 95.01461175692088545, -15.00000000000001421 ) ) ;
#16596=DIRECTION ( 'NONE',  ( 1.000000000000000000, 0.000000000000000000, 3.771137991253934490E-16 ) ) ;
#16598=CARTESIAN_POINT ( 'NONE',  ( -48.99724571598702738, 77.92691374209489652, 15.00000000000006928 ) ) ;
#16603=CARTESIAN_POINT ( 'NONE',  ( -68.94671286412481948, 88.15687341518439268, -167.1454815528550739 ) ) ;
#16609=VERTEX_POINT ( 'NONE', #3969 ) ;
#16610=CARTESIAN_POINT ( 'NONE',  ( -49.26569365422058411, 90.86016871721223254, 15.00000000000006928 ) ) ;
#16612=CARTESIAN_POINT ( 'NONE',  ( -57.08002265617300708, 84.22855780814606419, -15.00000000000001421 ) ) ;
#16614=ORIENTED_EDGE ( 'NONE', *, *, #5165, .F. ) ;
#16632=CARTESIAN_POINT ( 'NONE',  ( -64.58002265617299997, 84.22855780814606419, -15.00000000000001421 ) ) ;
#16635=CARTESIAN_POINT ( 'NONE',  ( -56.16856596726385220, 74.02016676429185793, 15.00000000000006928 ) ) ;
#16640=ADVANCED_FACE ( 'NONE', ( #8373 ), #8470, .T. ) ;
#16654=CYLINDRICAL_SURFACE ( 'NONE', #7232, 12.49999999999999645 ) ;
#16659=VECTOR ( 'NONE', #10045, 1000.000000000000000 ) ;
#16675=DIRECTION ( 'NONE',  ( 0.000000000000000000, 0.000000000000000000, 1.000000000000000000 ) ) ;
#16681=DIRECTION ( 'NONE',  ( 1.156482317317869999E-16, 0.000000000000000000, 1.000000000000000000 ) ) ;
#16685=DIRECTION ( 'NONE',  ( 1.000000000000000000, 0.000000000000000000, 5.551115123125786646E-16 ) ) ;
#16688=ORIENTED_EDGE ( 'NONE', *, *, #6885, .T. ) ;
#16691=EDGE_CURVE ( 'NONE', #5943, #4616, #8090, .T. ) ;
#16701=AXIS2_PLACEMENT_3D ( 'NONE', #3889, #18215, #12518 ) ;
#16703=DIRECTION ( 'NONE',  ( 1.156482317317869999E-16, 0.000000000000000000, 1.000000000000000000 ) ) ;
#16716=CARTESIAN_POINT ( 'NONE',  ( -63.25151023250651150, 93.09943318379590949, -167.1454815528550739 ) ) ;
#16723=DIRECTION ( 'NONE',  ( 1.000000000000000000, 0.000000000000000000, 5.551115123125774814E-16 ) ) ;
#16738=VECTOR ( 'NONE', #9150, 1000.000000000000000 ) ;
#16742=DIRECTION ( 'NONE',  ( 1.000000000000000000, 0.000000000000000000, 3.771137991253934490E-16 ) ) ;
#16752=VERTEX_POINT ( 'NONE', #5836 ) ;
#16758=CIRCLE ( 'NONE', #8713, 10.24900000000000055 ) ;
#16760=CARTESIAN_POINT ( 'NONE',  ( -47.13906347517657025, 79.99098546104539764, -167.1454815528550739 ) ) ;
#16773=VERTEX_POINT ( 'NONE', #17325 ) ;
#16777=EDGE_CURVE ( 'NONE', #4970, #9440, #16758, .T. ) ;
#16782=AXIS2_PLACEMENT_3D ( 'NONE', #3053, #1560, #16041 ) ;
#16784=LINE ( 'NONE', #16603, #8225 ) ;
#16786=AXIS2_PLACEMENT_3D ( 'NONE', #7441, #3314, #12897 ) ;
#16791=EDGE_CURVE ( 'NONE', #17079, #13750, #10199, .T. ) ;
#16794=ADVANCED_FACE ( 'NONE', ( #14273 ), #1539, .T. ) ;
#16799=CARTESIAN_POINT ( 'NONE',  ( -69.52933024547458274, 85.35316464920589397, -167.1454815528550739 ) ) ;
#16800=DIRECTION ( 'NONE',  ( 1.000000000000000000, 0.000000000000000000, 5.077734830647302671E-16 ) ) ;
#16802=DIRECTION ( 'NONE',  ( 1.156482317317869999E-16, 0.000000000000000000, 1.000000000000000000 ) ) ;
#16806=DIRECTION ( 'NONE',  ( 1.156482317317869999E-16, 0.000000000000000000, 1.000000000000000000 ) ) ;
#16816=DIRECTION ( 'NONE',  ( 1.156482317317869999E-16, 0.000000000000000000, 1.000000000000000000 ) ) ;
#16822=CIRCLE ( 'NONE', #8771, 4.599999999999992539 ) ;
#16824=CARTESIAN_POINT ( 'NONE',  ( -46.71322837820016360, 91.21279551874765446, 15.00000000000006928 ) ) ;
#16830=EDGE_LOOP ( 'NONE', ( #17602, #9346, #3177, #14851 ) ) ;
#16832=CARTESIAN_POINT ( 'NONE',  ( -57.08002265617300708, 84.22855780814606419, -167.1454815528550739 ) ) ;
#16833=CARTESIAN_POINT ( 'NONE',  ( -57.08002265617300708, 84.22855780814606419, -167.1454815528550739 ) ) ;
#16839=AXIS2_PLACEMENT_3D ( 'NONE', #6414, #12135, #10714 ) ;
#16840=DIRECTION ( 'NONE',  ( 1.000000000000000000, 0.000000000000000000, 3.771137991253928573E-16 ) ) ;
#16843=DIRECTION ( 'NONE',  ( -1.000000000000000000, -3.016910393003142859E-15, 0.000000000000000000 ) ) ;
#16850=DIRECTION ( 'NONE',  ( 1.156482317317869999E-16, 0.000000000000000000, 1.000000000000000000 ) ) ;
#16859=CARTESIAN_POINT ( 'NONE',  ( -45.39578445746348478, 88.67024416760654049, 15.00000000000009592 ) ) ;
#16860=CARTESIAN_POINT ( 'NONE',  ( -62.30871503255384170, 95.58244595420320877, -167.1454815528550739 ) ) ;
#16861=VERTEX_POINT ( 'NONE', #14703 ) ;
#16864=CIRCLE ( 'NONE', #13884, 4.599999999999999645 ) ;
#16868=ORIENTED_EDGE ( 'NONE', *, *, #14644, .F. ) ;
#16892=STYLED_ITEM('',(#18545),#12580);
#16893=VERTEX_POINT ( 'NONE', #3382 ) ;
#16898=ORIENTED_EDGE ( 'NONE', *, *, #17169, .F. ) ;
#16901=DIRECTION ( 'NONE',  ( 1.156482317317869999E-16, 0.000000000000000000, 1.000000000000000000 ) ) ;
#16903=DIRECTION ( 'NONE',  ( -1.000000000000000000, 0.000000000000000000, 0.000000000000000000 ) ) ;
#16907=DIRECTION ( 'NONE',  ( 0.000000000000000000, 0.000000000000000000, 1.000000000000000000 ) ) ;
#16909=CARTESIAN_POINT ( 'NONE',  ( -53.39175999306721110, 74.07097899412303832, -167.1454815528550739 ) ) ;
#16915=EDGE_CURVE ( 'NONE', #16085, #6741, #9919, .T. ) ;
#16916=CARTESIAN_POINT ( 'NONE',  ( -47.19781944808393348, 88.60139997190906058, -167.1454815528550739 ) ) ;
#16919=ORIENTED_EDGE ( 'NONE', *, *, #8334, .T. ) ;
#16921=ADVANCED_FACE ( 'NONE', ( #6466 ), #14800, .T. ) ;
#16923=DIRECTION ( 'NONE',  ( 1.000000000000000000, 0.000000000000000000, 0.000000000000000000 ) ) ;
#16928=ADVANCED_FACE ( 'NONE', ( #580 ), #9286, .T. ) ;
#16930=FACE_OUTER_BOUND ( 'NONE', #4195, .T. ) ;
#16933=EDGE_LOOP ( 'NONE', ( #11456, #17407, #18231, #9178 ) ) ;
#16940=DIRECTION ( 'NONE',  ( -1.000000000000000000, 6.033820786006295184E-15, 0.000000000000000000 ) ) ;
#16953=ORIENTED_EDGE ( 'NONE', *, *, #11231, .F. ) ;
#16957=DIRECTION ( 'NONE',  ( 1.000000000000000000, 0.000000000000000000, 5.077734830647302671E-16 ) ) ;
#16961=ORIENTED_EDGE ( 'NONE', *, *, #4678, .F. ) ;
#16963=VERTEX_POINT ( 'NONE', #15163 ) ;
#16967=CARTESIAN_POINT ( 'NONE',  ( -65.16279959635889441, 77.92691374209478283, 15.00000000000006928 ) ) ;
#16983=CYLINDRICAL_SURFACE ( 'NONE', #18041, 4.599999999999999645 ) ;
#16990=DIRECTION ( 'NONE',  ( 1.156482317317869999E-16, 0.000000000000000000, 1.000000000000000000 ) ) ;
#17004=ORIENTED_EDGE ( 'NONE', *, *, #12827, .T. ) ;
#17006=AXIS2_PLACEMENT_3D ( 'NONE', #2880, #16901, #14106 ) ;
#17015=DIRECTION ( 'NONE',  ( 1.156482317317869999E-16, 0.000000000000000000, 1.000000000000000000 ) ) ;
#17022=EDGE_CURVE ( 'NONE', #1931, #2889, #11423, .T. ) ;
#17023=CARTESIAN_POINT ( 'NONE',  ( -57.08002265617300708, 84.22855780814606419, -15.00000000000001421 ) ) ;
#17026=ORIENTED_EDGE ( 'NONE', *, *, #5852, .F. ) ;
#17028=ORIENTED_EDGE ( 'NONE', *, *, #13085, .F. ) ;
#17033=DIRECTION ( 'NONE',  ( 1.000000000000000000, 0.000000000000000000, 3.771137991253928573E-16 ) ) ;
#17034=ADVANCED_FACE ( 'NONE', ( #13969 ), #16654, .T. ) ;
#17037=DIRECTION ( 'NONE',  ( -1.000000000000000000, 0.000000000000000000, 0.000000000000000000 ) ) ;
#17041=VERTEX_POINT ( 'NONE', #6558 ) ;
#17043=DIRECTION ( 'NONE',  ( 1.156482317317869999E-16, 0.000000000000000000, 1.000000000000000000 ) ) ;
#17046=AXIS2_PLACEMENT_3D ( 'NONE', #1118, #16816, #9340 ) ;
#17054=ORIENTED_EDGE ( 'NONE', *, *, #17714, .F. ) ;
#17060=CIRCLE ( 'NONE', #5409, 12.50000000000000355 ) ;
#17066=ORIENTED_EDGE ( 'NONE', *, *, #10156, .T. ) ;
#17069=DIRECTION ( 'NONE',  ( 1.156482317317869999E-16, 0.000000000000000000, 1.000000000000000000 ) ) ;
#17075=EDGE_CURVE ( 'NONE', #13190, #8099, #14673, .T. ) ;
#17078=LINE ( 'NONE', #1184, #2523 ) ;
#17079=VERTEX_POINT ( 'NONE', #11598 ) ;
#17100=CARTESIAN_POINT ( 'NONE',  ( -53.53072411395612562, 94.43552448259771381, -15.00000000000001421 ) ) ;
#17104=EDGE_CURVE ( 'NONE', #15616, #14959, #6304, .T. ) ;
#17113=( LENGTH_UNIT ( ) NAMED_UNIT ( * ) SI_UNIT ( .MILLI., .METRE. ) );
#17124=ORIENTED_EDGE ( 'NONE', *, *, #13977, .F. ) ;
#17130=EDGE_CURVE ( 'NONE', #7016, #4262, #16160, .T. ) ;
#17138=VERTEX_POINT ( 'NONE', #10186 ) ;
#17141=ORIENTED_EDGE ( 'NONE', *, *, #3956, .F. ) ;
#17143=ORIENTED_EDGE ( 'NONE', *, *, #4232, .F. ) ;
#17159=VECTOR ( 'NONE', #10468, 1000.000000000000000 ) ;
#17164=VECTOR ( 'NONE', #7376, 1000.000000000000000 ) ;
#17168=ORIENTED_EDGE ( 'NONE', *, *, #16113, .F. ) ;
#17169=EDGE_CURVE ( 'NONE', #11983, #538, #3934, .T. ) ;
#17170=CIRCLE ( 'NONE', #9393, 4.599999999999999645 ) ;
#17176=DIRECTION ( 'NONE',  ( 0.000000000000000000, 0.000000000000000000, 1.000000000000000000 ) ) ;
#17179=EDGE_LOOP ( 'NONE', ( #16953, #16261, #15765, #12350 ) ) ;
#17181=CARTESIAN_POINT ( 'NONE',  ( -66.27474722583565381, 78.55081803573735044, -167.1454815528550739 ) ) ;
#17183=LINE ( 'NONE', #16799, #635 ) ;
#17193=DIRECTION ( 'NONE',  ( -5.204170427930409450E-16, 0.000000000000000000, 1.000000000000000000 ) ) ;
#17195=LINE ( 'NONE', #14023, #9884 ) ;
#17201=CIRCLE ( 'NONE', #465, 4.599999999999992539 ) ;
#17206=DIRECTION ( 'NONE',  ( 0.000000000000000000, 0.000000000000000000, 1.000000000000000000 ) ) ;
#17207=CARTESIAN_POINT ( 'NONE',  ( -50.90853507983961634, 93.09943318379598054, -15.00000000000001421 ) ) ;
#17210=ORIENTED_EDGE ( 'NONE', *, *, #5712, .T. ) ;
#17215=DIRECTION ( 'NONE',  ( 0.000000000000000000, 0.000000000000000000, 1.000000000000000000 ) ) ;
#17226=ORIENTED_EDGE ( 'NONE', *, *, #15148, .F. ) ;
#17227=DIRECTION ( 'NONE',  ( -1.000000000000000000, 0.000000000000000000, 1.387778780781446662E-16 ) ) ;
#17243=EDGE_CURVE ( 'NONE', #626, #10454, #3521, .T. ) ;
#17247=VERTEX_POINT ( 'NONE', #12336 ) ;
#17248=ORIENTED_EDGE ( 'NONE', *, *, #14201, .T. ) ;
#17250=ORIENTED_EDGE ( 'NONE', *, *, #14847, .F. ) ;
#17255=ADVANCED_FACE ( 'NONE', ( #10727 ), #18029, .T. ) ;
#17256=FACE_OUTER_BOUND ( 'NONE', #5797, .T. ) ;
#17258=DIRECTION ( 'NONE',  ( 0.000000000000000000, 0.000000000000000000, 1.000000000000000000 ) ) ;
#17261=ORIENTED_EDGE ( 'NONE', *, *, #13066, .F. ) ;
#17264=DIRECTION ( 'NONE',  ( 1.000000000000000000, 0.000000000000000000, 3.771137991253928573E-16 ) ) ;
#17270=EDGE_CURVE ( 'NONE', #9440, #2884, #7828, .T. ) ;
#17278=CYLINDRICAL_SURFACE ( 'NONE', #7045, 4.599999999999999645 ) ;
#17281=FACE_OUTER_BOUND ( 'NONE', #7617, .T. ) ;
#17287=CARTESIAN_POINT ( 'NONE',  ( -57.08002265617300708, 84.22855780814606419, 15.00000000000006928 ) ) ;
#17288=ORIENTED_EDGE ( 'NONE', *, *, #6287, .F. ) ;
#17289=ADVANCED_FACE ( 'NONE', ( #5494 ), #2796, .T. ) ;
#17291=LINE ( 'NONE', #14137, #6276 ) ;
#17298=ORIENTED_EDGE ( 'NONE', *, *, #440, .F. ) ;
#17303=DIRECTION ( 'NONE',  ( 1.000000000000000000, 0.000000000000000000, 0.000000000000000000 ) ) ;
#17306=DIRECTION ( 'NONE',  ( 0.000000000000000000, 0.000000000000000000, 1.000000000000000000 ) ) ;
#17311=DIRECTION ( 'NONE',  ( 1.000000000000000000, 0.000000000000000000, 0.000000000000000000 ) ) ;
#17312=CYLINDRICAL_SURFACE ( 'NONE', #16068, 12.50000000000000355 ) ;
#17325=CARTESIAN_POINT ( 'NONE',  ( -67.26033723204500347, 83.04399200740374454, 15.00000000000006928 ) ) ;
#17331=ORIENTED_EDGE ( 'NONE', *, *, #362, .F. ) ;
#17347=DIRECTION ( 'NONE',  ( -5.204170427930409450E-16, 0.000000000000000000, 1.000000000000000000 ) ) ;
#17352=CARTESIAN_POINT ( 'NONE',  ( -64.50972932340006594, 92.07579602767982863, -167.1454815528550739 ) ) ;
#17356=ORIENTED_EDGE ( 'NONE', *, *, #9161, .F. ) ;
#17360=CIRCLE ( 'NONE', #8430, 4.599999999999992539 ) ;
#17379=DIRECTION ( 'NONE',  ( 1.156482317317869999E-16, 0.000000000000000000, 1.000000000000000000 ) ) ;
#17382=ORIENTED_EDGE ( 'NONE', *, *, #440, .T. ) ;
#17388=CARTESIAN_POINT ( 'NONE',  ( -57.08002265617300708, 84.22855780814606419, -15.00000000000001421 ) ) ;
#17397=CYLINDRICAL_SURFACE ( 'NONE', #51, 12.50000000000001066 ) ;
#17399=CIRCLE ( 'NONE', #14699, 4.600000000000013856 ) ;
#17402=ORIENTED_EDGE ( 'NONE', *, *, #3791, .T. ) ;
#17407=ORIENTED_EDGE ( 'NONE', *, *, #7443, .T. ) ;
#17414=ORIENTED_EDGE ( 'NONE', *, *, #5626, .T. ) ;
#17421=CYLINDRICAL_SURFACE ( 'NONE', #1496, 4.599999999999999645 ) ;
#17422=ORIENTED_EDGE ( 'NONE', *, *, #17487, .F. ) ;
#17430=CLOSED_SHELL ( 'NONE', ( #14427, #9550, #7009, #1130, #11581, #2341, #12839, #5361, #16794, #1725, #6753, #2288, #1283, #5749, #13507, #1728, #17289, #9406, #3180, #8700, #2170, #14616, #13964, #1304, #7111, #9840, #13310, #1375, #7793, #1505, #7682, #16921, #16928, #15297, #12818, #14097, #11635, #16107, #8927, #9754, #2962, #4086, #15692, #16347, #20, #19, #1394, #11127, #12598, #14523, #340, #3493, #5639, #7439, #3116, #9476, #17505, #2382, #13509, #14536, #17034, #5595, #9828, #8812, #566, #7350, #16640, #17591, #2634, #13572, #9290, #1437, #13433, #7228, #12607, #11483, #12360, #14310, #6410, #9504, #12249, #15, #15565, #1249, #17255, #15956, #12381, #16019, #6382, #1256, #11082, #11531, #2551, #14985, #5912, #8723, #12622, #2773, #11338 ) ) ;
#17432=DIRECTION ( 'NONE',  ( -1.156482317317869999E-16, 0.000000000000000000, -1.000000000000000000 ) ) ;
#17444=FACE_OUTER_BOUND ( 'NONE', #2226, .T. ) ;
#17454=ORIENTED_EDGE ( 'NONE', *, *, #11897, .T. ) ;
#17461=CARTESIAN_POINT ( 'NONE',  ( -68.94671286412481948, 88.15687341518439268, -15.00000000000001243 ) ) ;
#17463=DIRECTION ( 'NONE',  ( -5.204170427930409450E-16, 0.000000000000000000, 1.000000000000000000 ) ) ;
#17465=CIRCLE ( 'NONE', #3412, 12.50000000000001066 ) ;
#17467=AXIS2_PLACEMENT_3D ( 'NONE', #16833, #6736, #16542 ) ;
#17472=DIRECTION ( 'NONE',  ( -5.204170427930409450E-16, 0.000000000000000000, 1.000000000000000000 ) ) ;
#17477=ORIENTED_EDGE ( 'NONE', *, *, #14970, .T. ) ;
#17479=CIRCLE ( 'NONE', #3157, 4.600000000000006750 ) ;
#17481=ORIENTED_EDGE ( 'NONE', *, *, #13282, .F. ) ;
#17482=DIRECTION ( 'NONE',  ( 1.000000000000000000, 0.000000000000000000, 5.077734830647302671E-16 ) ) ;
#17484=FACE_OUTER_BOUND ( 'NONE', #7071, .T. ) ;
#17485=DIRECTION ( 'NONE',  ( 0.000000000000000000, 0.000000000000000000, 1.000000000000000000 ) ) ;
#17487=EDGE_CURVE ( 'NONE', #9854, #16012, #71, .T. ) ;
#17499=CARTESIAN_POINT ( 'NONE',  ( -50.81952187608693805, 73.40930968350535579, 15.00000000000006928 ) ) ;
#17501=EDGE_CURVE ( 'NONE', #4498, #10224, #12010, .T. ) ;
#17502=EDGE_CURVE ( 'NONE', #4616, #16069, #8742, .T. ) ;
#17503=EDGE_CURVE ( 'NONE', #9222, #11275, #16477, .T. ) ;
#17505=ADVANCED_FACE ( 'NONE', ( #17444 ), #1826, .T. ) ;
#17506=CARTESIAN_POINT ( 'NONE',  ( -55.64822083176820655, 96.64628479562776420, -15.00000000000001421 ) ) ;
#17514=CARTESIAN_POINT ( 'NONE',  ( -44.78895386838529902, 81.95267818613812949, -167.1454815528550739 ) ) ;
#17515=ORIENTED_EDGE ( 'NONE', *, *, #6396, .F. ) ;
#17518=DIRECTION ( 'NONE',  ( -5.204170427930409450E-16, 0.000000000000000000, 1.000000000000000000 ) ) ;
#17530=DIRECTION ( 'NONE',  ( -5.204170427930409450E-16, 0.000000000000000000, 1.000000000000000000 ) ) ;
#17533=ORIENTED_EDGE ( 'NONE', *, *, #17022, .T. ) ;
#17535=CARTESIAN_POINT ( 'NONE',  ( -46.83322972390671879, 84.01587117655466841, -167.1454815528550739 ) ) ;
#17542=DIRECTION ( 'NONE',  ( 1.000000000000000000, 0.000000000000000000, 0.000000000000000000 ) ) ;
#17548=DIRECTION ( 'NONE',  ( -1.000000000000000000, 0.000000000000000000, 0.000000000000000000 ) ) ;
#17557=FACE_OUTER_BOUND ( 'NONE', #10244, .T. ) ;
#17558=LINE ( 'NONE', #6140, #18253 ) ;
#17559=ORIENTED_EDGE ( 'NONE', *, *, #10743, .T. ) ;
#17568=DIRECTION ( 'NONE',  ( 0.000000000000000000, 0.000000000000000000, 1.000000000000000000 ) ) ;
#17575=CIRCLE ( 'NONE', #11901, 10.24899999999998812 ) ;
#17581=ORIENTED_EDGE ( 'NONE', *, *, #12899, .T. ) ;
#17583=DIRECTION ( 'NONE',  ( -5.204170427930409450E-16, 0.000000000000000000, 1.000000000000000000 ) ) ;
#17584=AXIS2_PLACEMENT_3D ( 'NONE', #14589, #13715, #472 ) ;
#17591=ADVANCED_FACE ( 'NONE', ( #12208 ), #9411, .T. ) ;
#17595=EDGE_CURVE ( 'NONE', #5776, #70, #17979, .T. ) ;
#17601=CYLINDRICAL_SURFACE ( 'NONE', #849, 4.600000000000013856 ) ;
#17602=ORIENTED_EDGE ( 'NONE', *, *, #4335, .F. ) ;
#17603=AXIS2_PLACEMENT_3D ( 'NONE', #18198, #9689, #6690 ) ;
#17605=ORIENTED_EDGE ( 'NONE', *, *, #6889, .F. ) ;
#17610=EDGE_CURVE ( 'NONE', #11065, #12783, #1865, .T. ) ;
#17612=ORIENTED_EDGE ( 'NONE', *, *, #5852, .T. ) ;
#17618=CARTESIAN_POINT ( 'NONE',  ( -57.08002265617300708, 84.22855780814606419, 15.00000000000006928 ) ) ;
#17619=AXIS2_PLACEMENT_3D ( 'NONE', #12454, #14311, #8421 ) ;
#17623=DIRECTION ( 'NONE',  ( 1.000000000000000000, 0.000000000000000000, 5.551115123125786646E-16 ) ) ;
#17625=DIRECTION ( 'NONE',  ( -5.204170427930409450E-16, 0.000000000000000000, 1.000000000000000000 ) ) ;
#17650=CARTESIAN_POINT ( 'NONE',  ( -60.31105839772099841, 93.95493478196522119, -15.00000000000001421 ) ) ;
#17653=DIRECTION ( 'NONE',  ( -5.204170427930409450E-16, 0.000000000000000000, 1.000000000000000000 ) ) ;
#17655=ORIENTED_EDGE ( 'NONE', *, *, #12014, .T. ) ;
#17662=DIRECTION ( 'NONE',  ( 1.000000000000000000, 0.000000000000000000, 5.551115123125780730E-16 ) ) ;
#17673=AXIS2_PLACEMENT_3D ( 'NONE', #3503, #17900, #17623 ) ;
#17678=EDGE_LOOP ( 'NONE', ( #16174, #13365, #15265, #9572 ) ) ;
#17697=EDGE_CURVE ( 'NONE', #9204, #5292, #7843, .T. ) ;
#17699=EDGE_LOOP ( 'NONE', ( #220, #8433, #2568, #15248 ) ) ;
#17708=EDGE_CURVE ( 'NONE', #10347, #9500, #17399, .T. ) ;
#17709=EDGE_CURVE ( 'NONE', #4616, #5567, #2767, .T. ) ;
#17712=VECTOR ( 'NONE', #7726, 1000.000000000000000 ) ;
#17714=EDGE_CURVE ( 'NONE', #8377, #4219, #11446, .T. ) ;
#17717=ORIENTED_EDGE ( 'NONE', *, *, #8591, .F. ) ;
#17721=ORIENTED_EDGE ( 'NONE', *, *, #3956, .T. ) ;
#17732=ORIENTED_EDGE ( 'NONE', *, *, #13474, .F. ) ;
#17736=CIRCLE ( 'NONE', #3401, 10.24900000000000055 ) ;
#17742=DIRECTION ( 'NONE',  ( 0.000000000000000000, 0.000000000000000000, 1.000000000000000000 ) ) ;
#17744=DIRECTION ( 'NONE',  ( 1.156482317317869999E-16, 0.000000000000000000, 1.000000000000000000 ) ) ;
#17748=DIRECTION ( 'NONE',  ( 1.156482317317869999E-16, 0.000000000000000000, 1.000000000000000000 ) ) ;
#17750=ORIENTED_EDGE ( 'NONE', *, *, #17714, .T. ) ;
#17756=CARTESIAN_POINT ( 'NONE',  ( -46.89970808030100358, 83.04399200740388665, -167.1454815528550739 ) ) ;
#17759=DIRECTION ( 'NONE',  ( 0.000000000000000000, 0.000000000000000000, 1.000000000000000000 ) ) ;
#17763=VECTOR ( 'NONE', #3774, 1000.000000000000000 ) ;
#17781=EDGE_LOOP ( 'NONE', ( #6189, #12726, #4565, #6827 ) ) ;
#17782=DIRECTION ( 'NONE',  ( 1.156482317317869999E-16, 0.000000000000000000, 1.000000000000000000 ) ) ;
#17788=DIRECTION ( 'NONE',  ( 1.156482317317869999E-16, 0.000000000000000000, 1.000000000000000000 ) ) ;
#17790=AXIS2_PLACEMENT_3D ( 'NONE', #498, #7343, #10331 ) ;
#17794=CARTESIAN_POINT ( 'NONE',  ( -67.46561775476841660, 81.24207102880470188, -15.00000000000001421 ) ) ;
#17806=EDGE_CURVE ( 'NONE', #2040, #9854, #11289, .T. ) ;
#17808=CARTESIAN_POINT ( 'NONE',  ( -47.59681378869034774, 80.34130291867735707, 15.00000000000006928 ) ) ;
#17809=ORIENTED_EDGE ( 'NONE', *, *, #1831, .F. ) ;
#17810=CARTESIAN_POINT ( 'NONE',  ( -57.89103256796045116, 73.45256821284057480, 15.00000000000006928 ) ) ;
#17812=CYLINDRICAL_SURFACE ( 'NONE', #11426, 4.599999999999999645 ) ;
#17814=ORIENTED_EDGE ( 'NONE', *, *, #8486, .F. ) ;
#17824=DIRECTION ( 'NONE',  ( 0.000000000000000000, 0.000000000000000000, 1.000000000000000000 ) ) ;
#17826=ORIENTED_EDGE ( 'NONE', *, *, #13813, .T. ) ;
#17835=ORIENTED_EDGE ( 'NONE', *, *, #12951, .T. ) ;
#17838=EDGE_CURVE ( 'NONE', #8099, #12661, #10823, .T. ) ;
#17842=EDGE_CURVE ( 'NONE', #197, #11711, #8141, .T. ) ;
#17848=DIRECTION ( 'NONE',  ( 1.000000000000000000, 0.000000000000000000, 0.000000000000000000 ) ) ;
#17867=DIRECTION ( 'NONE',  ( 1.000000000000000000, 0.000000000000000000, 3.771137991253928573E-16 ) ) ;
#17869=CARTESIAN_POINT ( 'NONE',  ( -57.08002265617300708, 84.22855780814606419, -167.1454815528550739 ) ) ;
#17874=ORIENTED_EDGE ( 'NONE', *, *, #14291, .F. ) ;
#17880=EDGE_LOOP ( 'NONE', ( #13323, #2522, #6226, #12766 ) ) ;
#17886=EDGE_CURVE ( 'NONE', #1000, #18335, #673, .T. ) ;
#17889=CARTESIAN_POINT ( 'NONE',  ( -52.17699016282484337, 93.22868410554724505, -15.00000000000001421 ) ) ;
#17890=CARTESIAN_POINT ( 'NONE',  ( -57.08002265617300708, 84.22855780814606419, -167.1454815528550739 ) ) ;
#17900=DIRECTION ( 'NONE',  ( -5.204170427930409450E-16, 0.000000000000000000, 1.000000000000000000 ) ) ;
#17905=ORIENTED_EDGE ( 'NONE', *, *, #16102, .T. ) ;
#17918=ORIENTED_EDGE ( 'NONE', *, *, #11507, .T. ) ;
#17922=CARTESIAN_POINT ( 'NONE',  ( -57.08002265617300708, 84.22855780814606419, 15.00000000000006928 ) ) ;
#17924=CIRCLE ( 'NONE', #4777, 12.49999999999999645 ) ;
#17927=CIRCLE ( 'NONE', #7202, 12.50000000000000355 ) ;
#17928=EDGE_CURVE ( 'NONE', #14698, #16085, #9945, .T. ) ;
#17935=VERTEX_POINT ( 'NONE', #13673 ) ;
#17943=DIRECTION ( 'NONE',  ( 0.000000000000000000, 0.000000000000000000, 1.000000000000000000 ) ) ;
#17944=DIRECTION ( 'NONE',  ( 0.000000000000000000, 0.000000000000000000, 1.000000000000000000 ) ) ;
#17948=CYLINDRICAL_SURFACE ( 'NONE', #5141, 4.599999999999992539 ) ;
#17950=EDGE_CURVE ( 'NONE', #6278, #626, #14139, .T. ) ;
#17959=ORIENTED_EDGE ( 'NONE', *, *, #9537, .F. ) ;
#17966=CARTESIAN_POINT ( 'NONE',  ( -54.78701292294434211, 94.21775734381050427, -15.00000000000001421 ) ) ;
#17967=DIRECTION ( 'NONE',  ( -1.000000000000000000, 3.926781602367242350E-14, 1.692578276882432005E-16 ) ) ;
#17970=AXIS2_PLACEMENT_3D ( 'NONE', #514, #7907, #6298 ) ;
#17971=CARTESIAN_POINT ( 'NONE',  ( -63.16290507965269541, 75.97988867778799715, -15.00000000000001421 ) ) ;
#17976=DIRECTION ( 'NONE',  ( -1.000000000000000000, 5.107025913275718824E-14, 1.387778780781445182E-16 ) ) ;
#17979=CIRCLE ( 'NONE', #17673, 12.49999999999999112 ) ;
#18006=CIRCLE ( 'NONE', #8155, 7.500000000000000000 ) ;
#18015=ORIENTED_EDGE ( 'NONE', *, *, #5723, .F. ) ;
#18021=LINE ( 'NONE', #13541, #14716 ) ;
#18029=CYLINDRICAL_SURFACE ( 'NONE', #353, 12.49999999999999645 ) ;
#18041=AXIS2_PLACEMENT_3D ( 'NONE', #4173, #15694, #3983 ) ;
#18043=FACE_OUTER_BOUND ( 'NONE', #11908, .T. ) ;
#18062=EDGE_LOOP ( 'NONE', ( #17959, #3369, #1498, #4230 ) ) ;
#18072=EDGE_CURVE ( 'NONE', #9948, #3784, #14442, .T. ) ;
#18079=AXIS2_PLACEMENT_3D ( 'NONE', #10312, #13119, #4593 ) ;
#18080=DIRECTION ( 'NONE',  ( 1.156482317317869999E-16, 0.000000000000000000, 1.000000000000000000 ) ) ;
#18086=VECTOR ( 'NONE', #13262, 1000.000000000000000 ) ;
#18089=EDGE_CURVE ( 'NONE', #15247, #845, #16512, .T. ) ;
#18092=FACE_OUTER_BOUND ( 'NONE', #16159, .T. ) ;
#18095=ORIENTED_EDGE ( 'NONE', *, *, #3689, .T. ) ;
#18096=CIRCLE ( 'NONE', #14796, 4.599999999999992539 ) ;
#18098=CARTESIAN_POINT ( 'NONE',  ( -68.30128029835485393, 78.72098330317788850, 15.00000000000006928 ) ) ;
#18108=DIRECTION ( 'NONE',  ( 1.000000000000000000, 0.000000000000000000, 5.077734830647302671E-16 ) ) ;
#18113=ORIENTED_EDGE ( 'NONE', *, *, #8510, .F. ) ;
#18116=VERTEX_POINT ( 'NONE', #7576 ) ;
#18118=ORIENTED_EDGE ( 'NONE', *, *, #7237, .T. ) ;
#18123=DIRECTION ( 'NONE',  ( 0.000000000000000000, 0.000000000000000000, 1.000000000000000000 ) ) ;
#18124=DIRECTION ( 'NONE',  ( 0.000000000000000000, 0.000000000000000000, 1.000000000000000000 ) ) ;
#18126=DIRECTION ( 'NONE',  ( 1.000000000000000000, 0.000000000000000000, 0.000000000000000000 ) ) ;
#18130=CARTESIAN_POINT ( 'NONE',  ( -57.08002265617300708, 84.22855780814606419, -15.00000000000001421 ) ) ;
#18152=EDGE_LOOP ( 'NONE', ( #16614, #17612, #13346, #14429 ) ) ;
#18153=CARTESIAN_POINT ( 'NONE',  ( -47.88529808651028929, 78.55081803573747834, 15.00000000000006928 ) ) ;
#18155=ORIENTED_EDGE ( 'NONE', *, *, #8360, .T. ) ;
#18163=CARTESIAN_POINT ( 'NONE',  ( -51.34465738200551499, 92.72253132893560235, 15.00000000000006928 ) ) ;
#18164=CARTESIAN_POINT ( 'NONE',  ( -46.89970808030100358, 83.04399200740388665, -15.00000000000001421 ) ) ;
#18193=EDGE_LOOP ( 'NONE', ( #6437, #12793, #17477, #9195 ) ) ;
#18194=CYLINDRICAL_SURFACE ( 'NONE', #15570, 10.24899999999999345 ) ;
#18198=CARTESIAN_POINT ( 'NONE',  ( -61.98611128973170992, 74.59995546124152099, -15.00000000000001421 ) ) ;
#18199=DIRECTION ( 'NONE',  ( 0.000000000000000000, 0.000000000000000000, 1.000000000000000000 ) ) ;
#18201=EDGE_CURVE ( 'NONE', #1024, #1562, #5155, .T. ) ;
#18206=ORIENTED_EDGE ( 'NONE', *, *, #5730, .F. ) ;
#18215=DIRECTION ( 'NONE',  ( -5.204170427930409450E-16, 0.000000000000000000, 1.000000000000000000 ) ) ;
#18218=CIRCLE ( 'NONE', #17603, 4.600000000000006750 ) ;
#18221=CARTESIAN_POINT ( 'NONE',  ( -46.83322972390671879, 84.01587117655466841, 15.00000000000009592 ) ) ;
#18224=CARTESIAN_POINT ( 'NONE',  ( -57.08002265617300708, 84.22855780814606419, -15.00000000000001421 ) ) ;
#18225=CARTESIAN_POINT ( 'NONE',  ( -46.38449965345759551, 85.77305660501679085, 15.00000000000009592 ) ) ;
#18229=LINE ( 'NONE', #4617, #5986 ) ;
#18231=ORIENTED_EDGE ( 'NONE', *, *, #9537, .T. ) ;
#18234=VECTOR ( 'NONE', #14151, 1000.000000000000000 ) ;
#18235=DIRECTION ( 'NONE',  ( 1.000000000000000000, 0.000000000000000000, 0.000000000000000000 ) ) ;
#18236=CARTESIAN_POINT ( 'NONE',  ( -59.35080917176598092, 94.79374675277695417, -167.1454815528550739 ) ) ;
#18244=VECTOR ( 'NONE', #15528, 1000.000000000000000 ) ;
#18248=ORIENTED_EDGE ( 'NONE', *, *, #2552, .F. ) ;
#18249=CARTESIAN_POINT ( 'NONE',  ( -64.22944241949029731, 91.57211267264378307, -15.00000000000001421 ) ) ;
#18253=VECTOR ( 'NONE', #9162, 1000.000000000000000 ) ;
#18270=CARTESIAN_POINT ( 'NONE',  ( -66.56323152365561668, 80.34130291867722917, -15.00000000000001243 ) ) ;
#18271=DIRECTION ( 'NONE',  ( 0.000000000000000000, 0.000000000000000000, 1.000000000000000000 ) ) ;
#18275=CYLINDRICAL_SURFACE ( 'NONE', #1448, 4.600000000000006750 ) ;
#18277=EDGE_CURVE ( 'NONE', #11275, #9222, #18006, .T. ) ;
#18281=CARTESIAN_POINT ( 'NONE',  ( -48.98198201484814263, 93.75072866207695199, 15.00000000000006928 ) ) ;
#18282=CARTESIAN_POINT ( 'NONE',  ( -60.18936887439735273, 72.12145385653096241, 15.00000000000006928 ) ) ;
#18289=DIRECTION ( 'NONE',  ( 0.000000000000000000, 0.000000000000000000, 1.000000000000000000 ) ) ;
#18291=CARTESIAN_POINT ( 'NONE',  ( -57.08002265617300708, 84.22855780814606419, -167.1454815528550739 ) ) ;
#18298=ORIENTED_EDGE ( 'NONE', *, *, #11228, .T. ) ;
#18304=VECTOR ( 'NONE', #10552, 1000.000000000000000 ) ;
#18306=EDGE_CURVE ( 'NONE', #12513, #9457, #928, .T. ) ;
#18317=ORIENTED_EDGE ( 'NONE', *, *, #11231, .T. ) ;
#18320=CIRCLE ( 'NONE', #12658, 10.24900000000001477 ) ;
#18322=CARTESIAN_POINT ( 'NONE',  ( -57.08002265617300708, 84.22855780814606419, -167.1454815528550739 ) ) ;
#18330=AXIS2_PLACEMENT_3D ( 'NONE', #15878, #11673, #13351 ) ;
#18335=VERTEX_POINT ( 'NONE', #16351 ) ;
#18340=CARTESIAN_POINT ( 'NONE',  ( -45.21333244822126574, 88.15687341518456321, 15.00000000000006928 ) ) ;
#18355=CARTESIAN_POINT ( 'NONE',  ( -67.32681558843928826, 84.01587117655452630, -167.1454815528550739 ) ) ;
#18357=DIRECTION ( 'NONE',  ( -1.000000000000000000, 0.000000000000000000, 1.387778780781443703E-16 ) ) ;
#18359=VERTEX_POINT ( 'NONE', #6443 ) ;
#18360=ORIENTED_EDGE ( 'NONE', *, *, #3648, .F. ) ;
#18363=CARTESIAN_POINT ( 'NONE',  ( -68.05062368187118693, 78.23723799236674381, 15.00000000000006928 ) ) ;
#18367=LINE ( 'NONE', #2641, #7454 ) ;
#18377=CIRCLE ( 'NONE', #10587, 4.599999999999992539 ) ;
#18379=AXIS2_PLACEMENT_3D ( 'NONE', #9077, #15044, #10744 ) ;
#18384=AXIS2_PLACEMENT_3D ( 'NONE', #15834, #17583, #295 ) ;
#18386=AXIS2_PLACEMENT_3D ( 'NONE', #11846, #14560, #10258 ) ;
#18394=VERTEX_POINT ( 'NONE', #14033 ) ;
#18397=ORIENTED_EDGE ( 'NONE', *, *, #15790, .T. ) ;
#18408=ORIENTED_EDGE ( 'NONE', *, *, #18455, .F. ) ;
#18412=CARTESIAN_POINT ( 'NONE',  ( -51.34465738200551499, 92.72253132893560235, -167.1454815528550739 ) ) ;
#18427=VERTEX_POINT ( 'NONE', #18434 ) ;
#18431=LINE ( 'NONE', #439, #10853 ) ;
#18434=CARTESIAN_POINT ( 'NONE',  ( -51.81614838398844824, 95.01461175692088545, -15.00000000000001421 ) ) ;
#18438=EDGE_CURVE ( 'NONE', #11065, #13894, #5599, .T. ) ;
#18441=CARTESIAN_POINT ( 'NONE',  ( -57.08002265617300708, 84.22855780814606419, -15.00000000000001421 ) ) ;
#18455=EDGE_CURVE ( 'NONE', #1045, #9400, #4113, .T. ) ;
#18460=DIRECTION ( 'NONE',  ( -5.204170427930409450E-16, 0.000000000000000000, 1.000000000000000000 ) ) ;
#18462=DIRECTION ( 'NONE',  ( 1.000000000000000000, 0.000000000000000000, 0.000000000000000000 ) ) ;
#18473=FACE_OUTER_BOUND ( 'NONE', #17699, .T. ) ;
#18480=CARTESIAN_POINT ( 'NONE',  ( -57.08002265617300708, 84.22855780814606419, 15.00000000000006928 ) ) ;
#18489=VERTEX_POINT ( 'NONE', #86 ) ;
#18491=ORIENTED_EDGE ( 'NONE', *, *, #18089, .T. ) ;
#18498=DIRECTION ( 'NONE',  ( -5.204170427930409450E-16, 0.000000000000000000, 1.000000000000000000 ) ) ;
#18501=AXIS2_PLACEMENT_3D ( 'NONE', #8144, #12463, #16552 ) ;
#18504=ORIENTED_EDGE ( 'NONE', *, *, #4473, .F. ) ;
#18512=VECTOR ( 'NONE', #8627, 1000.000000000000000 ) ;
#18539=COLOUR_RGB('Light Blue',0.38,0.62,0.78);
#18540=FILL_AREA_STYLE_COLOUR('',#18539);
#18541=FILL_AREA_STYLE('',(#18540));
#18542=SURFACE_STYLE_FILL_AREA(#18541);
#18543=SURFACE_SIDE_STYLE('',(#18542));
#18544=SURFACE_STYLE_USAGE(.BOTH.,#18543);
#18545=PRESENTATION_STYLE_ASSIGNMENT((#18544));
ENDSEC;
END-ISO-10303-21;
